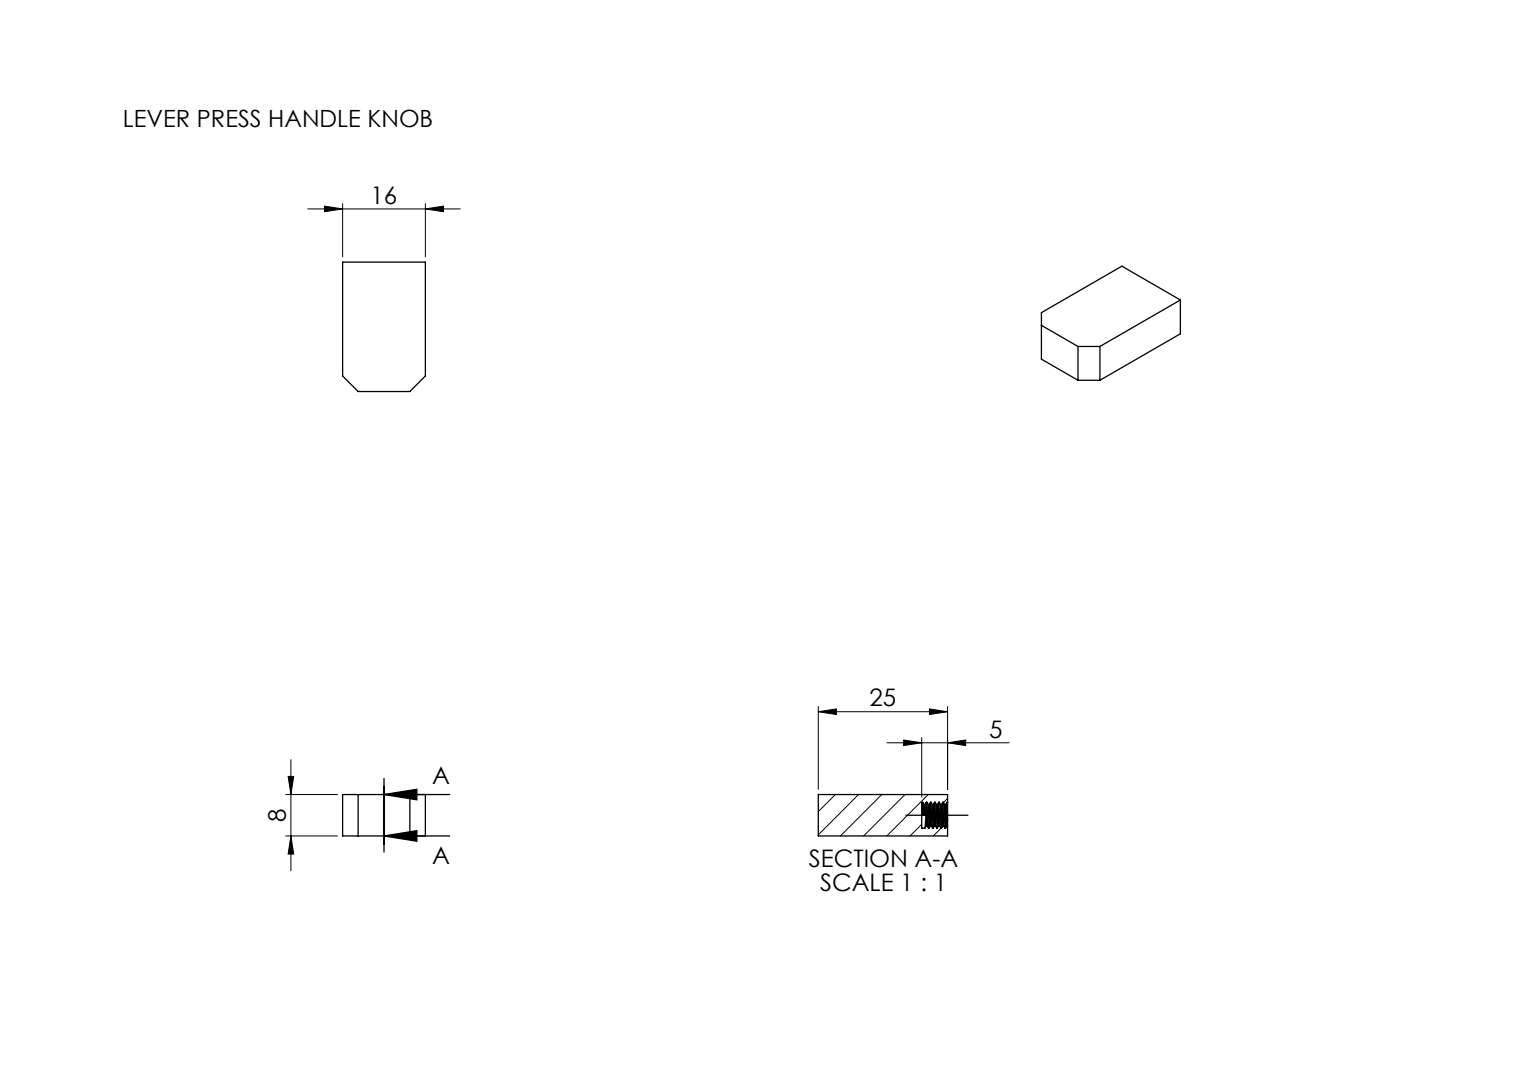
ISO-10303-21;
HEADER;
FILE_DESCRIPTION (('STEP AP214'),
    '1' );
FILE_NAME ('Lever Press Handle Knob.step',
    '2026-10-08T14:41:38',
    ( '' ),
    ( '' ),
    'SwSTEP 2.0',
    'SolidWorks 2026',
    '' );
FILE_SCHEMA (( 'AUTOMOTIVE_DESIGN' ));
ENDSEC;

DATA;
#12=LINE ( 'NONE', #3049, #2216 ) ;
#27=MECHANICAL_DESIGN_GEOMETRIC_PRESENTATION_REPRESENTATION('',(#18516),#10981);
#30=CARTESIAN_POINT ( 'NONE',  ( 2.500000000000001776, 64.00000000000000000, 49.99999999999999289 ) ) ;
#45=CARTESIAN_POINT ( 'NONE',  ( 4.592425496802577917E-16, 61.50000000000000000, 46.19999999999999574 ) ) ;
#69=CARTESIAN_POINT ( 'NONE',  ( 2.066987300000001859, 63.14382582708704916, 46.10000000109246798 ) ) ;
#77=ORIENTED_EDGE ( 'NONE', *, *, #16848, .F. ) ;
#82=CARTESIAN_POINT ( 'NONE',  ( 2.500000000000006661, 65.03553390593272354, 48.04999999999999716 ) ) ;
#83=CARTESIAN_POINT ( 'NONE',  ( 2.066987300000001859, 64.85617417291294373, 46.80000000109246372 ) ) ;
#85=EDGE_LOOP ( 'NONE', ( #12730, #3911, #462, #6972, #16450, #10959, #3705, #8319, #7529, #13845, #6781, #19380, #3029, #10375 ) ) ;
#92=CARTESIAN_POINT ( 'NONE',  ( -2.066987300000001415, 63.14382582708705627, 46.60000000109246088 ) ) ;
#105=CARTESIAN_POINT ( 'NONE',  ( 2.500000000000002220, 62.96446609406726225, 47.25000000218494023 ) ) ;
#113=DIRECTION ( 'NONE',  ( -0.000000000000000000, -0.000000000000000000, -1.000000000000000000 ) ) ;
#135=CARTESIAN_POINT ( 'NONE',  ( 0.000000000000000000, 64.00000000000000000, 49.99999999999999289 ) ) ;
#139=CARTESIAN_POINT ( 'NONE',  ( -2.500000000000001776, 64.00000000000000000, 46.79999999999999716 ) ) ;
#140=CARTESIAN_POINT ( 'NONE',  ( 4.592425496802577917E-16, 61.50000000000000000, 46.99999999999999289 ) ) ;
#161=CARTESIAN_POINT ( 'NONE',  ( 1.461580736456473906, 62.53841926354353120, 45.25000000109247367 ) ) ;
#162=CARTESIAN_POINT ( 'NONE',  ( -1.461580736456473906, 65.46158073645646880, 49.65000000109246514 ) ) ;
#179=DIRECTION ( 'NONE',  ( -0.000000000000000000, -0.000000000000000000, -1.000000000000000000 ) ) ;
#180=CARTESIAN_POINT ( 'NONE',  ( -2.066987300000001415, 64.00000000000000000, 46.35000000109246798 ) ) ;
#188=CARTESIAN_POINT ( 'NONE',  ( 2.066987300000001859, 64.85617417291294373, 46.20000000109247651 ) ) ;
#189=EDGE_CURVE ( 'NONE', #14847, #7431, #12616, .T. ) ;
#229=CARTESIAN_POINT ( 'NONE',  ( 1.767766952966369987, 65.76776695296638309, 45.69999999999999574 ) ) ;
#245=CARTESIAN_POINT ( 'NONE',  ( -0.8996865886453131456, 66.25031470727165583, 44.99999999999998579 ) ) ;
#257=CARTESIAN_POINT ( 'NONE',  ( -2.066987300000001415, 63.14382582708705627, 47.40000000109247225 ) ) ;
#270=CARTESIAN_POINT ( 'NONE',  ( 2.066987300000001415, 64.00000000000000000, 47.55000000109247082 ) ) ;
#271=ORIENTED_EDGE ( 'NONE', *, *, #18253, .T. ) ;
#278=CARTESIAN_POINT ( 'NONE',  ( -2.066987300000000971, 63.14382582708704916, 48.00000000109246656 ) ) ;
#296=CARTESIAN_POINT ( 'NONE',  ( 1.767766952966370653, 62.23223304703363112, 47.20000000218494307 ) ) ;
#316=CARTESIAN_POINT ( 'NONE',  ( 2.500000000000001776, 64.00000000000000000, 46.50000000218494733 ) ) ;
#331=AXIS2_PLACEMENT_3D ( 'NONE', #17063, #3625, #15585 ) ;
#334=LINE ( 'NONE', #13649, #1223 ) ;
#335=DIRECTION ( 'NONE',  ( -1.000000000000000000, 0.000000000000000000, 0.000000000000000000 ) ) ;
#345=AXIS2_PLACEMENT_3D ( 'NONE', #135, #15137, #1704 ) ;
#360=CARTESIAN_POINT ( 'NONE',  ( -1.265664690411616068E-16, 66.06698730000000808, 46.35000000109246798 ) ) ;
#373=CARTESIAN_POINT ( 'NONE',  ( -2.500000000000001776, 64.00000000000000000, 48.39999999999999858 ) ) ;
#374=CARTESIAN_POINT ( 'NONE',  ( 3.796994071234847710E-16, 61.93301269999999903, 47.35000000109246798 ) ) ;
#380=DIRECTION ( 'NONE',  ( -0.000000000000000000, -0.000000000000000000, -1.000000000000000000 ) ) ;
#382=CARTESIAN_POINT ( 'NONE',  ( -2.066987300000001415, 64.85617417291294373, 49.50000000109246656 ) ) ;
#385=CARTESIAN_POINT ( 'NONE',  ( 0.8561741729129460632, 66.06698729999999387, 45.50000000109247367 ) ) ;
#388=CARTESIAN_POINT ( 'NONE',  ( 2.500000000000001776, 64.00000000000000000, 47.30000000218494449 ) ) ;
#390=EDGE_LOOP ( 'NONE', ( #5193, #765, #2617, #19104 ) ) ;
#391=EDGE_LOOP ( 'NONE', ( #18321, #5980, #17279, #6106, #2334 ) ) ;
#405=CARTESIAN_POINT ( 'NONE',  ( 2.500000000000001776, 64.00000000000000000, 45.59999999999999432 ) ) ;
#410=CARTESIAN_POINT ( 'NONE',  ( 0.8561741729129472844, 61.93301270000000613, 48.20000000109248361 ) ) ;
#429=LINE ( 'NONE', #4946, #12185 ) ;
#438=CARTESIAN_POINT ( 'NONE',  ( -2.500000000000001776, 64.00000000000000000, 47.70000000218494307 ) ) ;
#455=CARTESIAN_POINT ( 'NONE',  ( -1.461580736456473906, 65.46158073645646880, 48.05000000109247082 ) ) ;
#462=ORIENTED_EDGE ( 'NONE', *, *, #8308, .F. ) ;
#467=CARTESIAN_POINT ( 'NONE',  ( -2.066987300000001859, 64.85617417291294373, 47.90000000109247225 ) ) ;
#470=CARTESIAN_POINT ( 'NONE',  ( -2.500000000000011546, 65.03553390593272354, 46.05000000218494449 ) ) ;
#473=CARTESIAN_POINT ( 'NONE',  ( 3.796994071234847710E-16, 61.93301269999999903, 48.95000000109246940 ) ) ;
#481=EDGE_LOOP ( 'NONE', ( #15484, #1248, #5355, #15133 ) ) ;
#491=DIRECTION ( 'NONE',  ( -1.000000000000000000, -0.000000000000000000, -0.000000000000000000 ) ) ;
#531=CARTESIAN_POINT ( 'NONE',  ( 1.767766952966369987, 65.76776695296638309, 46.49999999999999289 ) ) ;
#535=VERTEX_POINT ( 'NONE', #8772 ) ;
#548=DIRECTION ( 'NONE',  ( -1.000000000000000000, 0.000000000000000000, 0.000000000000000000 ) ) ;
#550=CARTESIAN_POINT ( 'NONE',  ( -1.265664690411616068E-16, 66.06698730000000808, 47.15000000109247225 ) ) ;
#566=CARTESIAN_POINT ( 'NONE',  ( -2.066987300000001415, 64.85617417291294373, 47.90000000109247225 ) ) ;
#568=LINE ( 'NONE', #6369, #960 ) ;
#574=VERTEX_POINT ( 'NONE', #10335 ) ;
#581=VECTOR ( 'NONE', #2799, 1000.000000000000000 ) ;
#595=CARTESIAN_POINT ( 'NONE',  ( 0.8561741729129460632, 66.06698729999999387, 47.70000000109248361 ) ) ;
#597=CARTESIAN_POINT ( 'NONE',  ( -2.066987300000000971, 63.14382582708704916, 48.20000000109247651 ) ) ;
#623=CARTESIAN_POINT ( 'NONE',  ( -1.767766952966370209, 65.76776695296638309, 45.09999999999999432 ) ) ;
#637=FACE_OUTER_BOUND ( 'NONE', #1554, .T. ) ;
#647=CARTESIAN_POINT ( 'NONE',  ( -0.8561741729129465073, 61.93301270000000613, 48.30000000109247082 ) ) ;
#663=VERTEX_POINT ( 'NONE', #14958 ) ;
#669=CARTESIAN_POINT ( 'NONE',  ( 2.066987300000001859, 63.14382582708704916, 49.10000000109246088 ) ) ;
#677=VERTEX_POINT ( 'NONE', #10628 ) ;
#680=( NAMED_UNIT ( * ) PLANE_ANGLE_UNIT ( ) SI_UNIT ( $, .RADIAN. ) );
#682=ORIENTED_EDGE ( 'NONE', *, *, #6769, .F. ) ;
#683=EDGE_LOOP ( 'NONE', ( #8801, #8791, #6089, #8526 ) ) ;
#687=CARTESIAN_POINT ( 'NONE',  ( 2.500000000000001776, 64.00000000000000000, 47.30000000218494449 ) ) ;
#699=LINE ( 'NONE', #15785, #15320 ) ;
#700=CARTESIAN_POINT ( 'NONE',  ( -1.265664690411616068E-16, 66.06698730000000808, 48.55000000109247082 ) ) ;
#701=CARTESIAN_POINT ( 'NONE',  ( -2.066987300000001415, 64.85617417291294373, 49.70000000109247651 ) ) ;
#740=CARTESIAN_POINT ( 'NONE',  ( -2.500000000000001776, 64.00000000000000000, 48.50000000218494023 ) ) ;
#741=CARTESIAN_POINT ( 'NONE',  ( 2.066987300000001859, 64.85617417291294373, 46.20000000109247651 ) ) ;
#753=CARTESIAN_POINT ( 'NONE',  ( -0.8561741729129466183, 61.93301270000000613, 45.70000000109248361 ) ) ;
#761=CARTESIAN_POINT ( 'NONE',  ( -2.499999999999998668, 62.96446609406726225, 47.64999999999999858 ) ) ;
#765=ORIENTED_EDGE ( 'NONE', *, *, #8549, .F. ) ;
#772=CARTESIAN_POINT ( 'NONE',  ( -2.500000000000001776, 64.00000000000000000, 48.50000000218494023 ) ) ;
#784=CARTESIAN_POINT ( 'NONE',  ( 2.066987300000002303, 63.14382582708705627, 45.10000000109246798 ) ) ;
#786=CARTESIAN_POINT ( 'NONE',  ( 1.461580736456473906, 62.53841926354353120, 48.45000000109246940 ) ) ;
#812=DIRECTION ( 'NONE',  ( 0.7071067811865463515, 0.000000000000000000, -0.7071067811865487940 ) ) ;
#832=CARTESIAN_POINT ( 'NONE',  ( -2.500000000000000888, 62.96446609406726935, 48.44999999999999574 ) ) ;
#839=CARTESIAN_POINT ( 'NONE',  ( 2.500000000000001776, 64.00000000000000000, 48.79999999999999716 ) ) ;
#845=CARTESIAN_POINT ( 'NONE',  ( -1.265664690411616068E-16, 66.06698730000000808, 46.95000000109246940 ) ) ;
#847=EDGE_CURVE ( 'NONE', #14186, #5501, #5607, .T. ) ;
#863=CARTESIAN_POINT ( 'NONE',  ( -1.530808498934192803E-16, 66.50000000000000000, 49.10000000218494165 ) ) ;
#875=CARTESIAN_POINT ( 'NONE',  ( -1.461580736456473906, 65.46158073645646880, 47.05000000109247082 ) ) ;
#879=LINE ( 'NONE', #8340, #1099 ) ;
#907=ADVANCED_FACE ( 'NONE', ( #15824 ), #16023, .F. ) ;
#926=CARTESIAN_POINT ( 'NONE',  ( 2.500000000000002220, 62.96446609406726935, 49.54999999999999716 ) ) ;
#942=CARTESIAN_POINT ( 'NONE',  ( 2.066987300000001415, 64.00000000000000000, 47.55000000109247082 ) ) ;
#957=EDGE_CURVE ( 'NONE', #15953, #1682, #18392, .T. ) ;
#960=VECTOR ( 'NONE', #4995, 1000.000000000000000 ) ;
#962=CARTESIAN_POINT ( 'NONE',  ( -1.767766952966369765, 62.23223304703363112, 47.00000000218494733 ) ) ;
#976=CARTESIAN_POINT ( 'NONE',  ( 2.066987300000001415, 64.00000000000000000, 45.95000000109246940 ) ) ;
#980=CARTESIAN_POINT ( 'NONE',  ( 1.145374997815830520, 62.22070308213160672, 44.99999999999998579 ) ) ;
#986=ORIENTED_EDGE ( 'NONE', *, *, #5520, .T. ) ;
#994=CIRCLE ( 'NONE', #16652, 2.500000000000001776 ) ;
#1004=CARTESIAN_POINT ( 'NONE',  ( -2.066987300000001415, 64.00000000000000000, 49.55000000109247082 ) ) ;
#1028=CARTESIAN_POINT ( 'NONE',  ( 1.035533905932738197, 66.50000000000000000, 48.94999999999999574 ) ) ;
#1040=CARTESIAN_POINT ( 'NONE',  ( 2.066987300000001859, 63.14382582708704916, 45.90000000109247225 ) ) ;
#1055=CARTESIAN_POINT ( 'NONE',  ( 1.035533905932738197, 66.50000000000000000, 46.65000000218494591 ) ) ;
#1067=CARTESIAN_POINT ( 'NONE',  ( 3.796994071234847710E-16, 61.93301269999999903, 46.55000000109247082 ) ) ;
#1099=VECTOR ( 'NONE', #2541, 1000.000000000000000 ) ;
#1104=CARTESIAN_POINT ( 'NONE',  ( -1.265664690411616068E-16, 66.06698730000000808, 44.55000000109247082 ) ) ;
#1120=CARTESIAN_POINT ( 'NONE',  ( 2.066987300000001859, 64.85617417291294373, 45.40000000109246514 ) ) ;
#1136=CARTESIAN_POINT ( 'NONE',  ( -2.066987300000001415, 64.00000000000000000, 46.35000000109246798 ) ) ;
#1139=CARTESIAN_POINT ( 'NONE',  ( 2.066987300000001859, 63.14382582708704916, 47.70000000109246940 ) ) ;
#1154=CARTESIAN_POINT ( 'NONE',  ( 0.8561741729129472844, 61.93301270000000613, 49.00000000109246656 ) ) ;
#1164=CARTESIAN_POINT ( 'NONE',  ( 0.8561741729129460632, 66.06698729999999387, 46.90000000109247225 ) ) ;
#1194=DIRECTION ( 'NONE',  ( -1.000000000000000000, 0.000000000000000000, 0.000000000000000000 ) ) ;
#1210=EDGE_CURVE ( 'NONE', #9690, #15813, #699, .T. ) ;
#1213=CARTESIAN_POINT ( 'NONE',  ( 2.500000000000002220, 62.96446609406726935, 45.54999999999999716 ) ) ;
#1223=VECTOR ( 'NONE', #16705, 1000.000000000000000 ) ;
#1234=CARTESIAN_POINT ( 'NONE',  ( -2.066987300000001415, 64.00000000000000000, 48.95000000109246940 ) ) ;
#1248=ORIENTED_EDGE ( 'NONE', *, *, #14177, .T. ) ;
#1255=CARTESIAN_POINT ( 'NONE',  ( -1.035533905932738863, 61.50000000000000000, 45.45000000218495018 ) ) ;
#1259=VERTEX_POINT ( 'NONE', #9699 ) ;
#1266=CARTESIAN_POINT ( 'NONE',  ( 2.066987300000002303, 63.14382582708705627, 48.50000000109246656 ) ) ;
#1323=CARTESIAN_POINT ( 'NONE',  ( -2.500000000000001776, 65.03553390593273775, 45.14999999999999858 ) ) ;
#1330=CARTESIAN_POINT ( 'NONE',  ( -2.169199425089220146, 64.10592246629431656, 45.00000000000000000 ) ) ;
#1347=SHAPE_REPRESENTATION_RELATIONSHIP ( 'NONE' , 'NONE' ,  #15288, #12018 ) ;
#1355=CARTESIAN_POINT ( 'NONE',  ( 1.767766952966369987, 65.76776695296638309, 45.80000000218493739 ) ) ;
#1367=CARTESIAN_POINT ( 'NONE',  ( 3.796994071234847710E-16, 61.93301269999999903, 47.55000000109247082 ) ) ;
#1387=CARTESIAN_POINT ( 'NONE',  ( 8.000000000000014211, 60.00000000000000711, 45.00000000000000000 ) ) ;
#1396=ORIENTED_EDGE ( 'NONE', *, *, #6504, .F. ) ;
#1417=CARTESIAN_POINT ( 'NONE',  ( 4.592425496802577917E-16, 61.50000000000000000, 47.79999999999999716 ) ) ;
#1437=CARTESIAN_POINT ( 'NONE',  ( -2.066987300000001415, 64.85617417291294373, 45.70000000109248361 ) ) ;
#1454=CARTESIAN_POINT ( 'NONE',  ( 4.592425496802577917E-16, 61.50000000000000000, 44.70000000218494307 ) ) ;
#1466=CARTESIAN_POINT ( 'NONE',  ( -2.066987300000001415, 63.14382582708705627, 47.40000000109247225 ) ) ;
#1470=CARTESIAN_POINT ( 'NONE',  ( -7.999999999999986677, 68.00000000000000000, 66.99999999999997158 ) ) ;
#1477=ORIENTED_EDGE ( 'NONE', *, *, #18253, .F. ) ;
#1494=CARTESIAN_POINT ( 'NONE',  ( -2.499999999999992006, 62.96446609406726225, 46.15000000218496012 ) ) ;
#1508=ORIENTED_EDGE ( 'NONE', *, *, #15852, .T. ) ;
#1519=CARTESIAN_POINT ( 'NONE',  ( 1.035533905932738197, 66.50000000000000000, 47.34999999999999432 ) ) ;
#1521=ORIENTED_EDGE ( 'NONE', *, *, #17939, .T. ) ;
#1526=CARTESIAN_POINT ( 'NONE',  ( -1.909647267044692676, 63.20899822134837365, 45.00000000000000000 ) ) ;
#1540=ORIENTED_EDGE ( 'NONE', *, *, #6380, .F. ) ;
#1552=CARTESIAN_POINT ( 'NONE',  ( 0.8561741729129460632, 66.06698729999999387, 49.30000000109246372 ) ) ;
#1554=EDGE_LOOP ( 'NONE', ( #9866, #4096, #2330, #1508, #682, #6069 ) ) ;
#1561=CARTESIAN_POINT ( 'NONE',  ( -0.8561741729129465073, 61.93301270000000613, 46.70000000109248361 ) ) ;
#1588=FACE_OUTER_BOUND ( 'NONE', #481, .T. ) ;
#1604=CARTESIAN_POINT ( 'NONE',  ( -2.500000000000001776, 64.00000000000000000, 47.70000000218494307 ) ) ;
#1621=CARTESIAN_POINT ( 'NONE',  ( -1.530808498934192803E-16, 66.50000000000000000, 48.19999999999999574 ) ) ;
#1642=CARTESIAN_POINT ( 'NONE',  ( -2.066987300000001415, 64.00000000000000000, 46.55000000109247082 ) ) ;
#1645=FACE_OUTER_BOUND ( 'NONE', #683, .T. ) ;
#1656=CARTESIAN_POINT ( 'NONE',  ( 3.796994071234847710E-16, 61.93301269999999903, 48.15000000109247225 ) ) ;
#1660=CARTESIAN_POINT ( 'NONE',  ( 1.767766952966369987, 65.76776695296638309, 45.80000000218493739 ) ) ;
#1665=CARTESIAN_POINT ( 'NONE',  ( 2.066987300000002303, 63.14382582708705627, 46.90000000109247225 ) ) ;
#1667=CARTESIAN_POINT ( 'NONE',  ( -1.767766952966370209, 65.76776695296638309, 47.60000000218494165 ) ) ;
#1682=VERTEX_POINT ( 'NONE', #9102 ) ;
#1687=CARTESIAN_POINT ( 'NONE',  ( -2.500000000000001776, 64.00000000000000000, 46.10000000218494165 ) ) ;
#1704=DIRECTION ( 'NONE',  ( -1.000000000000000000, 0.000000000000000000, 0.000000000000000000 ) ) ;
#1731=CARTESIAN_POINT ( 'NONE',  ( 0.8561741729129471734, 61.93301270000000613, 46.00000000109246656 ) ) ;
#1732=CARTESIAN_POINT ( 'NONE',  ( -0.8561741729129465073, 61.93301270000000613, 46.70000000109248361 ) ) ;
#1733=DIRECTION ( 'NONE',  ( -0.7071067811865463515, 0.000000000000000000, -0.7071067811865487940 ) ) ;
#1747=CARTESIAN_POINT ( 'NONE',  ( 1.461580736456473684, 65.46158073645646880, 46.85000000109246798 ) ) ;
#1754=FACE_OUTER_BOUND ( 'NONE', #4883, .T. ) ;
#1791=AXIS2_PLACEMENT_3D ( 'NONE', #13713, #4815, #7646 ) ;
#1816=EDGE_CURVE ( 'NONE', #6405, #8644, #12331, .T. ) ;
#1827=DIRECTION ( 'NONE',  ( -0.000000000000000000, -0.000000000000000000, -1.000000000000000000 ) ) ;
#1828=CARTESIAN_POINT ( 'NONE',  ( -1.530808498934192803E-16, 66.50000000000000000, 48.30000000218494449 ) ) ;
#1829=CARTESIAN_POINT ( 'NONE',  ( 3.796994071234847710E-16, 61.93301269999999903, 49.15000000109246514 ) ) ;
#1841=CARTESIAN_POINT ( 'NONE',  ( -2.066987300000001859, 64.85617417291294373, 46.30000000109247082 ) ) ;
#1855=CARTESIAN_POINT ( 'NONE',  ( -1.035533905932738863, 61.50000000000000000, 45.45000000218494307 ) ) ;
#1886=CARTESIAN_POINT ( 'NONE',  ( 0.000000000000000000, 64.00000000000000000, 49.99999999999999289 ) ) ;
#1897=( BOUNDED_CURVE ( )  B_SPLINE_CURVE ( 2, ( #3126, #18429, #1667, #13901, #3522, #10664, #16664, #3229, #388 ),
 .UNSPECIFIED., .F., .F. ) 
 B_SPLINE_CURVE_WITH_KNOTS ( ( 3, 2, 2, 2, 3 ),
 ( 0.2857142857142859205, 0.3035714285714287142, 0.3214285714285715634, 0.3392857142857143571, 0.3571428571428571508 ),
 .UNSPECIFIED. ) 
 CURVE ( )  GEOMETRIC_REPRESENTATION_ITEM ( )  RATIONAL_B_SPLINE_CURVE ( ( 0.9999999999999990008, 0.9238795325112877377, 1.000000000000000000, 0.9238795325112867385, 1.000000000000000000, 0.9238795325112867385, 1.000000000000000000, 0.9238795325112867385, 1.000000000000000000 ) ) 
 REPRESENTATION_ITEM ( '' )  );
#1933=CARTESIAN_POINT ( 'NONE',  ( -1.461580736456473906, 65.46158073645646880, 48.85000000109246798 ) ) ;
#1935=ORIENTED_EDGE ( 'NONE', *, *, #14860, .F. ) ;
#1946=CARTESIAN_POINT ( 'NONE',  ( 2.066987300000001415, 64.00000000000000000, 45.95000000109246940 ) ) ;
#1953=CARTESIAN_POINT ( 'NONE',  ( 1.461580736456473906, 62.53841926354353120, 45.25000000109247367 ) ) ;
#1961=ORIENTED_EDGE ( 'NONE', *, *, #10797, .F. ) ;
#1980=CARTESIAN_POINT ( 'NONE',  ( -1.461580736456473906, 65.46158073645646880, 48.65000000109247225 ) ) ;
#2014=CARTESIAN_POINT ( 'NONE',  ( 2.499999999999996891, 62.96446609406726225, 47.14999999999999147 ) ) ;
#2020=CARTESIAN_POINT ( 'NONE',  ( -2.066987300000001415, 64.00000000000000000, 47.35000000109246798 ) ) ;
#2030=CARTESIAN_POINT ( 'NONE',  ( 0.7910017786515960436, 62.09035273295529578, 44.99999999999998579 ) ) ;
#2033=CARTESIAN_POINT ( 'NONE',  ( -0.8561741729129461742, 66.06698729999999387, 47.00000000109247367 ) ) ;
#2037=CARTESIAN_POINT ( 'NONE',  ( 2.500000000000001776, 65.03553390593273775, 45.75000000218494733 ) ) ;
#2063=( NAMED_UNIT ( * ) SI_UNIT ( $, .STERADIAN. ) SOLID_ANGLE_UNIT ( ) );
#2066=ORIENTED_EDGE ( 'NONE', *, *, #14389, .F. ) ;
#2114=CARTESIAN_POINT ( 'NONE',  ( -1.767766952966369765, 62.23223304703363112, 46.89999999999999858 ) ) ;
#2121=CARTESIAN_POINT ( 'NONE',  ( 1.461580736456473906, 62.53841926354353120, 46.85000000109246798 ) ) ;
#2138=CARTESIAN_POINT ( 'NONE',  ( -2.500000000000001776, 64.00000000000000000, 49.99999999999999289 ) ) ;
#2139=CARTESIAN_POINT ( 'NONE',  ( -1.461580736456473906, 65.46158073645646880, 44.85000000109246798 ) ) ;
#2140=FACE_OUTER_BOUND ( 'NONE', #5028, .T. ) ;
#2152=CARTESIAN_POINT ( 'NONE',  ( -2.500000000000000888, 62.96446609406726935, 47.75000000218494023 ) ) ;
#2156=PRESENTATION_STYLE_ASSIGNMENT (( #12547 ) ) ;
#2165=CARTESIAN_POINT ( 'NONE',  ( 1.461580736456473684, 65.46158073645646880, 47.05000000109247082 ) ) ;
#2183=CARTESIAN_POINT ( 'NONE',  ( -2.500000000000001776, 64.00000000000000000, 45.30000000218493739 ) ) ;
#2200=VECTOR ( 'NONE', #3797, 1000.000000000000000 ) ;
#2211=CARTESIAN_POINT ( 'NONE',  ( -7.999999999999986677, 60.00000000000000711, 45.00000000000000000 ) ) ;
#2214=CARTESIAN_POINT ( 'NONE',  ( 1.767766952966370653, 62.23223304703363112, 48.69999999999999574 ) ) ;
#2216=VECTOR ( 'NONE', #9024, 1000.000000000000000 ) ;
#2232=CARTESIAN_POINT ( 'NONE',  ( -1.265664690411616068E-16, 66.06698730000000808, 45.35000000109246798 ) ) ;
#2240=ORIENTED_EDGE ( 'NONE', *, *, #2551, .T. ) ;
#2251=CARTESIAN_POINT ( 'NONE',  ( -2.500000000000001776, 65.03553390593273775, 49.25000000218494023 ) ) ;
#2263=CARTESIAN_POINT ( 'NONE',  ( 2.066987300000001415, 64.00000000000000000, 49.15000000109247225 ) ) ;
#2264=CARTESIAN_POINT ( 'NONE',  ( 0.8561741729129471734, 61.93301270000000613, 46.80000000109247082 ) ) ;
#2287=CARTESIAN_POINT ( 'NONE',  ( 11.00000000000002309, 68.00000000000000000, 63.99999999999994316 ) ) ;
#2293=EDGE_CURVE ( 'NONE', #6744, #15813, #4783, .T. ) ;
#2300=CARTESIAN_POINT ( 'NONE',  ( 2.500000000000001776, 64.00000000000000000, 46.50000000218494733 ) ) ;
#2305=CARTESIAN_POINT ( 'NONE',  ( 1.035533905932739751, 61.50000000000000000, 49.44999999999999574 ) ) ;
#2328=CARTESIAN_POINT ( 'NONE',  ( -1.035533905932738863, 61.50000000000000000, 47.74999999999999289 ) ) ;
#2330=ORIENTED_EDGE ( 'NONE', *, *, #15528, .F. ) ;
#2334=ORIENTED_EDGE ( 'NONE', *, *, #9822, .F. ) ;
#2341=CARTESIAN_POINT ( 'NONE',  ( -2.500000000000001776, 64.00000000000000000, 46.10000000218494165 ) ) ;
#2348=CARTESIAN_POINT ( 'NONE',  ( -1.909647267044692676, 63.20899822134837365, 45.00000000000000000 ) ) ;
#2351=CARTESIAN_POINT ( 'NONE',  ( -1.265664690411616068E-16, 66.06698730000000808, 49.55000000109247082 ) ) ;
#2353=CARTESIAN_POINT ( 'NONE',  ( -2.066987300000001415, 64.00000000000000000, 47.35000000109246798 ) ) ;
#2362=VERTEX_POINT ( 'NONE', #14169 ) ;
#2396=CARTESIAN_POINT ( 'NONE',  ( 1.035533905932738197, 66.50000000000000000, 49.75000000000000000 ) ) ;
#2410=CARTESIAN_POINT ( 'NONE',  ( -2.066987300000001415, 64.85617417291294373, 47.10000000109246798 ) ) ;
#2427=CARTESIAN_POINT ( 'NONE',  ( 2.500000000000002220, 62.96446609406726935, 48.05000000218494449 ) ) ;
#2440=CARTESIAN_POINT ( 'NONE',  ( 0.8561741729129472844, 61.93301270000000613, 46.60000000109246088 ) ) ;
#2443=CARTESIAN_POINT ( 'NONE',  ( 1.976658868803501834, 62.97126298013989754, 45.00000000000001421 ) ) ;
#2476=CARTESIAN_POINT ( 'NONE',  ( -2.066987300000001859, 64.85617417291294373, 44.70000000109248361 ) ) ;
#2482=CARTESIAN_POINT ( 'NONE',  ( 2.499999999999999112, 65.03553390593273775, 46.55000000218494449 ) ) ;
#2489=CARTESIAN_POINT ( 'NONE',  ( -2.066987300000001415, 63.14382582708705627, 45.80000000109246372 ) ) ;
#2506=CARTESIAN_POINT ( 'NONE',  ( 2.066987300000001415, 64.85617417291294373, 46.00000000109247367 ) ) ;
#2525=CARTESIAN_POINT ( 'NONE',  ( -2.500000000000000888, 62.96446609406726935, 46.95000000218495018 ) ) ;
#2537=CARTESIAN_POINT ( 'NONE',  ( 0.8561741729129460632, 66.06698729999999387, 46.10000000109246798 ) ) ;
#2541=DIRECTION ( 'NONE',  ( -0.7071067811865463515, 0.000000000000000000, 0.7071067811865487940 ) ) ;
#2551=EDGE_CURVE ( 'NONE', #10838, #14706, #8107, .T. ) ;
#2564=CARTESIAN_POINT ( 'NONE',  ( -2.283493650000001818, 64.00000000000000000, 49.87500000054622973 ) ) ;
#2568=DIRECTION ( 'NONE',  ( -0.8660254037844385966, 0.000000000000000000, 0.5000000000000001110 ) ) ;
#2576=CARTESIAN_POINT ( 'NONE',  ( -0.8561741729129465073, 61.93301270000000613, 44.90000000109247225 ) ) ;
#2588=CARTESIAN_POINT ( 'NONE',  ( 0.8561741729129472844, 61.93301270000000613, 46.00000000109245946 ) ) ;
#2601=CARTESIAN_POINT ( 'NONE',  ( -2.066987300000000971, 63.14382582708704916, 45.60000000109246798 ) ) ;
#2610=ORIENTED_EDGE ( 'NONE', *, *, #17643, .F. ) ;
#2615=CARTESIAN_POINT ( 'NONE',  ( 0.8561741729129472844, 61.93301270000000613, 48.20000000109248361 ) ) ;
#2617=ORIENTED_EDGE ( 'NONE', *, *, #13137, .F. ) ;
#2626=CARTESIAN_POINT ( 'NONE',  ( 2.066987300000001859, 64.85617417291294373, 45.20000000109248361 ) ) ;
#2645=EDGE_CURVE ( 'NONE', #677, #16168, #16710, .T. ) ;
#2688=CARTESIAN_POINT ( 'NONE',  ( -1.767766952966369765, 62.23223304703363112, 45.29999999999999005 ) ) ;
#2705=CARTESIAN_POINT ( 'NONE',  ( 2.066987300000001415, 64.00000000000000000, 46.95000000109246940 ) ) ;
#2706=DIRECTION ( 'NONE',  ( 0.7071067811865487940, 1.226634733346701480E-15, 0.7071067811865462405 ) ) ;
#2721=CARTESIAN_POINT ( 'NONE',  ( -1.767766952966369765, 62.23223304703363112, 45.40000000218494591 ) ) ;
#2732=CARTESIAN_POINT ( 'NONE',  ( -2.066987300000001415, 64.00000000000000000, 49.75000000109246656 ) ) ;
#2779=CARTESIAN_POINT ( 'NONE',  ( -2.500000000000001776, 65.03553390593273775, 46.74999999999999289 ) ) ;
#2780=CARTESIAN_POINT ( 'NONE',  ( 1.035533905932739751, 61.50000000000000000, 46.24999999999998579 ) ) ;
#2786=EDGE_CURVE ( 'NONE', #18046, #15953, #15628, .T. ) ;
#2799=DIRECTION ( 'NONE',  ( 0.000000000000000000, 0.000000000000000000, 1.000000000000000000 ) ) ;
#2800=DIRECTION ( 'NONE',  ( -1.000000000000000000, 0.000000000000000000, 0.000000000000000000 ) ) ;
#2802=CARTESIAN_POINT ( 'NONE',  ( -1.461580736456473906, 65.46158073645646880, 48.85000000109246798 ) ) ;
#2806=ORIENTED_EDGE ( 'NONE', *, *, #19318, .F. ) ;
#2818=CARTESIAN_POINT ( 'NONE',  ( -2.500000000000001776, 65.03553390593273775, 46.05000000218494449 ) ) ;
#2828=CARTESIAN_POINT ( 'NONE',  ( 0.8561741729129472844, 61.93301270000000613, 47.60000000109246798 ) ) ;
#2847=DIRECTION ( 'NONE',  ( -1.000000000000000000, 0.000000000000000000, 0.000000000000000000 ) ) ;
#2848=ORIENTED_EDGE ( 'NONE', *, *, #957, .F. ) ;
#2882=CARTESIAN_POINT ( 'NONE',  ( -1.767766952966370209, 65.76776695296638309, 47.49999999999999289 ) ) ;
#2904=CARTESIAN_POINT ( 'NONE',  ( -0.8561741729129461742, 66.06698729999999387, 49.60000000109246798 ) ) ;
#2918=CARTESIAN_POINT ( 'NONE',  ( -1.265664690411616068E-16, 66.06698730000000808, 48.55000000109247082 ) ) ;
#2926=CARTESIAN_POINT ( 'NONE',  ( -0.8561741729129461742, 66.06698729999999387, 48.80000000109247082 ) ) ;
#2927=EDGE_CURVE ( 'NONE', #3230, #15072, #9595, .T. ) ;
#2951=DIRECTION ( 'NONE',  ( -0.000000000000000000, -0.000000000000000000, -1.000000000000000000 ) ) ;
#2953=CARTESIAN_POINT ( 'NONE',  ( -1.035533905932738863, 61.50000000000000000, 46.25000000218494733 ) ) ;
#2963=CARTESIAN_POINT ( 'NONE',  ( -1.530808498934192803E-16, 66.50000000000000000, 45.79999999999999005 ) ) ;
#2973=FACE_OUTER_BOUND ( 'NONE', #9281, .T. ) ;
#2976=CARTESIAN_POINT ( 'NONE',  ( 1.767766952966370653, 62.23223304703363112, 47.89999999999999858 ) ) ;
#2983=CARTESIAN_POINT ( 'NONE',  ( -0.1886580908559672143, 66.48422237085870279, 45.00000000000000711 ) ) ;
#2995=DIRECTION ( 'NONE',  ( 0.8660254037844385966, 0.000000000000000000, 0.5000000000000001110 ) ) ;
#2996=CARTESIAN_POINT ( 'NONE',  ( 2.066987300000001415, 64.00000000000000000, 45.35000000109246798 ) ) ;
#3011=CARTESIAN_POINT ( 'NONE',  ( -1.767766952966369765, 62.23223304703363112, 48.60000000218494165 ) ) ;
#3015=CARTESIAN_POINT ( 'NONE',  ( -1.767766952966370209, 65.76776695296638309, 44.40000000218493881 ) ) ;
#3020=ORIENTED_EDGE ( 'NONE', *, *, #8179, .F. ) ;
#3025=CARTESIAN_POINT ( 'NONE',  ( 2.066987300000001415, 64.00000000000000000, 47.75000000109246656 ) ) ;
#3029=ORIENTED_EDGE ( 'NONE', *, *, #17851, .T. ) ;
#3030=ORIENTED_EDGE ( 'NONE', *, *, #15550, .T. ) ;
#3043=ADVANCED_FACE ( 'NONE', ( #14207 ), #10769, .T. ) ;
#3046=ORIENTED_EDGE ( 'NONE', *, *, #10797, .T. ) ;
#3049=CARTESIAN_POINT ( 'NONE',  ( 8.000000000000000000, 68.00000000000000000, 45.00000000000000000 ) ) ;
#3075=CARTESIAN_POINT ( 'NONE',  ( 2.500000000000001776, 64.00000000000000000, 47.99999999999999289 ) ) ;
#3076=CARTESIAN_POINT ( 'NONE',  ( -2.500000000000001776, 64.00000000000000000, 49.99999999999999289 ) ) ;
#3094=CARTESIAN_POINT ( 'NONE',  ( -1.461580736456473462, 62.53841926354353120, 46.65000000109247225 ) ) ;
#3109=CARTESIAN_POINT ( 'NONE',  ( 2.500000000000001776, 64.00000000000000000, 48.90000000218494591 ) ) ;
#3114=CARTESIAN_POINT ( 'NONE',  ( 2.066987300000001415, 64.00000000000000000, 46.75000000109247367 ) ) ;
#3123=CARTESIAN_POINT ( 'NONE',  ( 0.8561741729129460632, 66.06698729999999387, 46.30000000109247082 ) ) ;
#3126=CARTESIAN_POINT ( 'NONE',  ( -2.500000000000001776, 64.00000000000000000, 47.70000000218494307 ) ) ;
#3149=CARTESIAN_POINT ( 'NONE',  ( -2.500000000000001776, 64.00000000000000000, 49.99999999999999289 ) ) ;
#3162=ORIENTED_EDGE ( 'NONE', *, *, #13703, .F. ) ;
#3180=DIRECTION ( 'NONE',  ( 1.000000000000000000, 0.000000000000000000, -0.000000000000000000 ) ) ;
#3184=EDGE_CURVE ( 'NONE', #10801, #17922, #3906, .T. ) ;
#3196=CARTESIAN_POINT ( 'NONE',  ( -7.999999999999986677, 60.00000000000000711, 45.00000000000000000 ) ) ;
#3203=CARTESIAN_POINT ( 'NONE',  ( 2.066987300000001415, 64.00000000000000000, 46.15000000109247225 ) ) ;
#3208=ORIENTED_EDGE ( 'NONE', *, *, #12727, .T. ) ;
#3219=CARTESIAN_POINT ( 'NONE',  ( -2.066987300000001415, 63.14382582708705627, 45.60000000109246088 ) ) ;
#3225=CARTESIAN_POINT ( 'NONE',  ( 2.066987300000001415, 64.85617417291294373, 48.40000000109247225 ) ) ;
#3227=CARTESIAN_POINT ( 'NONE',  ( 1.461580736456473906, 62.53841926354353120, 46.05000000109246372 ) ) ;
#3229=CARTESIAN_POINT ( 'NONE',  ( 2.500000000000001776, 65.03553390593273775, 47.35000000218494165 ) ) ;
#3230=VERTEX_POINT ( 'NONE', #17522 ) ;
#3245=CARTESIAN_POINT ( 'NONE',  ( -2.499999999999996003, 62.96446609406726225, 45.25000000000000000 ) ) ;
#3250=DIRECTION ( 'NONE',  ( -0.000000000000000000, -0.000000000000000000, -1.000000000000000000 ) ) ;
#3255=ADVANCED_FACE ( 'NONE', ( #11528 ), #8258, .F. ) ;
#3297=EDGE_CURVE ( 'NONE', #574, #8644, #10230, .T. ) ;
#3302=CARTESIAN_POINT ( 'NONE',  ( 1.767766952966369987, 65.76776695296638309, 48.20000000218494307 ) ) ;
#3303=CARTESIAN_POINT ( 'NONE',  ( -1.265664690411616068E-16, 66.06698730000000808, 47.95000000109246940 ) ) ;
#3317=CARTESIAN_POINT ( 'NONE',  ( -2.500000000000001776, 64.00000000000000000, 49.99999999999999289 ) ) ;
#3318=CARTESIAN_POINT ( 'NONE',  ( 1.461580736456473684, 65.46158073645646880, 45.25000000109247367 ) ) ;
#3323=ORIENTED_EDGE ( 'NONE', *, *, #13137, .T. ) ;
#3337=ORIENTED_EDGE ( 'NONE', *, *, #1816, .F. ) ;
#3355=CARTESIAN_POINT ( 'NONE',  ( 1.461580736456473906, 62.53841926354353120, 49.05000000109247082 ) ) ;
#3376=LINE ( 'NONE', #3076, #14576 ) ;
#3392=CARTESIAN_POINT ( 'NONE',  ( -2.066987300000001859, 64.85617417291294373, 48.10000000109246798 ) ) ;
#3407=CARTESIAN_POINT ( 'NONE',  ( -2.066987300000001415, 64.00000000000000000, 47.15000000109247225 ) ) ;
#3408=ORIENTED_EDGE ( 'NONE', *, *, #1816, .T. ) ;
#3413=CARTESIAN_POINT ( 'NONE',  ( -1.265664690411616068E-16, 66.06698730000000808, 48.55000000109247082 ) ) ;
#3415=CARTESIAN_POINT ( 'NONE',  ( -0.8561741729129465073, 61.93301270000000613, 45.10000000109246798 ) ) ;
#3452=ORIENTED_EDGE ( 'NONE', *, *, #14948, .F. ) ;
#3473=CARTESIAN_POINT ( 'NONE',  ( -1.530808498934192803E-16, 66.50000000000000000, 45.00000000000000000 ) ) ;
#3476=ORIENTED_EDGE ( 'NONE', *, *, #6386, .F. ) ;
#3490=DIRECTION ( 'NONE',  ( 0.000000000000000000, 0.000000000000000000, 1.000000000000000000 ) ) ;
#3493=CARTESIAN_POINT ( 'NONE',  ( -1.461580736456473462, 62.53841926354353120, 47.45000000109246230 ) ) ;
#3511=CARTESIAN_POINT ( 'NONE',  ( -1.461580736456473906, 65.46158073645646880, 46.25000000109247367 ) ) ;
#3515=CARTESIAN_POINT ( 'NONE',  ( 1.035533905932738197, 66.50000000000000000, 45.85000000218494165 ) ) ;
#3519=EDGE_CURVE ( 'NONE', #7431, #4122, #10990, .T. ) ;
#3520=CARTESIAN_POINT ( 'NONE',  ( -1.461580736456473906, 65.46158073645646880, 45.65000000109247225 ) ) ;
#3522=CARTESIAN_POINT ( 'NONE',  ( -1.530808498934192803E-16, 66.50000000000000000, 47.50000000218494023 ) ) ;
#3536=EDGE_CURVE ( 'NONE', #5700, #574, #13446, .T. ) ;
#3544=CARTESIAN_POINT ( 'NONE',  ( -1.461580736456473906, 65.46158073645646880, 47.85000000109246798 ) ) ;
#3586=CARTESIAN_POINT ( 'NONE',  ( 1.461580736456473906, 62.53841926354353120, 49.25000000109246656 ) ) ;
#3597=CARTESIAN_POINT ( 'NONE',  ( 3.796994071234847710E-16, 61.93301269999999903, 44.95000000109246940 ) ) ;
#3605=CARTESIAN_POINT ( 'NONE',  ( -1.461580736456473906, 65.46158073645646880, 49.45000000109246940 ) ) ;
#3624=CARTESIAN_POINT ( 'NONE',  ( -1.035533905932738641, 66.50000000000000000, 49.15000000218494591 ) ) ;
#3625=DIRECTION ( 'NONE',  ( 1.000000000000000000, 1.734723475976807094E-15, -0.000000000000000000 ) ) ;
#3630=VERTEX_POINT ( 'NONE', #9435 ) ;
#3637=CARTESIAN_POINT ( 'NONE',  ( -2.066987300000001859, 64.85617417291294373, 48.70000000109247651 ) ) ;
#3638=VECTOR ( 'NONE', #15142, 1000.000000000000000 ) ;
#3639=CARTESIAN_POINT ( 'NONE',  ( -1.461580736456473906, 65.46158073645646880, 47.25000000109246656 ) ) ;
#3642=CARTESIAN_POINT ( 'NONE',  ( -1.530808498934192803E-16, 66.50000000000000000, 45.00000000000000000 ) ) ;
#3658=CARTESIAN_POINT ( 'NONE',  ( -1.530808498934192803E-16, 66.50000000000000000, 45.10000000218494165 ) ) ;
#3666=LINE ( 'NONE', #6616, #3950 ) ;
#3672=MECHANICAL_DESIGN_GEOMETRIC_PRESENTATION_REPRESENTATION('',(#5247),#6190);
#3675=DIRECTION ( 'NONE',  ( 0.000000000000000000, -0.000000000000000000, 1.000000000000000000 ) ) ;
#3684=CARTESIAN_POINT ( 'NONE',  ( 0.8561741729129472844, 61.93301270000000613, 47.60000000109246798 ) ) ;
#3698=CARTESIAN_POINT ( 'NONE',  ( -2.066987300000001415, 64.85617417291294373, 45.50000000109247367 ) ) ;
#3702=CARTESIAN_POINT ( 'NONE',  ( -7.999999999999986677, 68.00000000000000000, 66.99999999999997158 ) ) ;
#3705=ORIENTED_EDGE ( 'NONE', *, *, #10956, .T. ) ;
#3707=( LENGTH_UNIT ( ) NAMED_UNIT ( * ) SI_UNIT ( .MILLI., .METRE. ) );
#3715=CARTESIAN_POINT ( 'NONE',  ( 2.500000000000001776, 64.00000000000000000, 48.90000000218494591 ) ) ;
#3723=CARTESIAN_POINT ( 'NONE',  ( 0.5387381024323600887, 61.98586169951557423, 44.99999999999999289 ) ) ;
#3727=CARTESIAN_POINT ( 'NONE',  ( -1.461580736456473462, 62.53841926354353120, 47.25000000109247367 ) ) ;
#3728=CARTESIAN_POINT ( 'NONE',  ( -1.265664690411616068E-16, 66.06698730000000808, 48.75000000109246656 ) ) ;
#3729=CARTESIAN_POINT ( 'NONE',  ( -4.999999999999980460, 60.00000000000000711, 69.99999999999998579 ) ) ;
#3762=UNCERTAINTY_MEASURE_WITH_UNIT (LENGTH_MEASURE( 1.000000000000000082E-05 ), #3707, 'distance_accuracy_value', 'NONE');
#3774=CARTESIAN_POINT ( 'NONE',  ( 1.767766952966369987, 65.76776695296638309, 46.60000000218494165 ) ) ;
#3783=CARTESIAN_POINT ( 'NONE',  ( -0.8561741729129461742, 66.06698729999999387, 44.80000000109246372 ) ) ;
#3797=DIRECTION ( 'NONE',  ( -0.000000000000000000, -0.000000000000000000, -1.000000000000000000 ) ) ;
#3800=CARTESIAN_POINT ( 'NONE',  ( 2.066987300000001415, 64.00000000000000000, 45.15000000109247225 ) ) ;
#3802=CARTESIAN_POINT ( 'NONE',  ( -2.500000000000001776, 64.00000000000000000, 49.30000000218494449 ) ) ;
#3816=CARTESIAN_POINT ( 'NONE',  ( -1.035533905932738863, 61.50000000000000000, 46.25000000218494733 ) ) ;
#3817=DIRECTION ( 'NONE',  ( 0.000000000000000000, 0.000000000000000000, 1.000000000000000000 ) ) ;
#3823=CARTESIAN_POINT ( 'NONE',  ( -1.366300952416055425, 62.44303698707672368, 45.00000000000000711 ) ) ;
#3826=CARTESIAN_POINT ( 'NONE',  ( -0.8561741729129461742, 66.06698729999999387, 44.60000000109246088 ) ) ;
#3827=CARTESIAN_POINT ( 'NONE',  ( -0.8561741729129461742, 66.06698730000000808, 49.60000000109247509 ) ) ;
#3870=CARTESIAN_POINT ( 'NONE',  ( -1.265664690411616068E-16, 66.06698730000000808, 45.55000000109246372 ) ) ;
#3891=ADVANCED_FACE ( 'NONE', ( #7656 ), #13622, .T. ) ;
#3905=CARTESIAN_POINT ( 'NONE',  ( -1.767766952966370209, 65.76776695296638309, 49.20000000218494307 ) ) ;
#3906=LINE ( 'NONE', #8325, #8745 ) ;
#3911=ORIENTED_EDGE ( 'NONE', *, *, #5520, .F. ) ;
#3915=CARTESIAN_POINT ( 'NONE',  ( -0.8561741729129465073, 61.93301270000000613, 44.90000000109247225 ) ) ;
#3920=CARTESIAN_POINT ( 'NONE',  ( 2.154726813346381942, 63.29944981661203229, 45.00000000000002842 ) ) ;
#3950=VECTOR ( 'NONE', #12672, 1000.000000000000000 ) ;
#3958=MANIFOLD_SOLID_BREP ( 'Cavity1', #7554 ) ;
#3969=CARTESIAN_POINT ( 'NONE',  ( 1.767766952966369987, 65.76776695296638309, 49.69999999999999574 ) ) ;
#3977=CARTESIAN_POINT ( 'NONE',  ( -1.767766952966370209, 65.76776695296638309, 49.09999999999999432 ) ) ;
#3983=CARTESIAN_POINT ( 'NONE',  ( 0.8561741729129460632, 66.06698730000000808, 46.10000000109246798 ) ) ;
#4000=CARTESIAN_POINT ( 'NONE',  ( 2.500000000000002220, 62.96446609406726935, 47.25000000218494023 ) ) ;
#4010=CARTESIAN_POINT ( 'NONE',  ( -2.066987300000001415, 63.14382582708705627, 46.40000000109246514 ) ) ;
#4013=CARTESIAN_POINT ( 'NONE',  ( -2.500000000000003553, 62.96446609406726225, 49.24999999999997868 ) ) ;
#4032=AXIS2_PLACEMENT_3D ( 'NONE', #13057, #15738, #11490 ) ;
#4047=CARTESIAN_POINT ( 'NONE',  ( -1.035533905932738863, 61.50000000000000000, 48.54999999999999716 ) ) ;
#4062=CARTESIAN_POINT ( 'NONE',  ( -1.767766952966370209, 65.76776695296638309, 49.89999999999999147 ) ) ;
#4078=CARTESIAN_POINT ( 'NONE',  ( 2.066987300000001859, 63.14382582708704916, 46.70000000109248361 ) ) ;
#4096=ORIENTED_EDGE ( 'NONE', *, *, #6380, .T. ) ;
#4101=CARTESIAN_POINT ( 'NONE',  ( 2.066987300000002303, 63.14382582708705627, 48.30000000109247082 ) ) ;
#4114=CARTESIAN_POINT ( 'NONE',  ( -0.8561741729129461742, 66.06698729999999387, 49.60000000109246798 ) ) ;
#4122=VERTEX_POINT ( 'NONE', #11530 ) ;
#4124=( BOUNDED_SURFACE ( )  B_SPLINE_SURFACE ( 1, 2, ( 
 ( #9701, #12358, #8063, #9418, #14125, #12266, #11167, #6490, #2263, #6589, #3355, #12454, #6682, #4928, #4831, #15412, #7867, #3637, #1980, #16783, #700, #9320, #7963, #14217, #5022, #5124, #10980, #410, #13928, #10885, #16880, #16985, #12556, #6395, #3544, #18356, #14023, #595, #11077, #17075, #9609, #15595, #12647, #18645, #5212, #17166, #3727, #15693, #6296, #10072, #875, #14309, #9884, #1164, #17440, #15974, #7141, #6854, #9973, #2440, #1067, #18733, #11256, #4010, #4209, #8334, #6952, #19014, #5484, #2537, #12827, #8520, #976, #11447, #13109, #5298, #9793, #8423, #15786, #11538, #17258, #18824, #5579, #12737, #14494, #17347, #16066, #2626, #5398, #784, #17536, #19109, #11354, #3915, #7044, #15878, #14595, #16162, #6771, #3826, #13014 ),
 ( #2732, #10161, #11642, #4114, #2351, #5682, #14399, #8611, #17633, #18917, #8703, #12923, #16458, #5873, #10661, #16556, #14688, #9103, #8904, #2926, #4706, #12036, #11835, #7243, #15092, #1266, #10369, #16662, #7435, #13512, #14891, #16255, #17832, #13305, #19305, #4408, #14986, #14796, #16363, #13214, #3025, #4308, #13403, #2828, #1367, #9002, #19205, #1466, #7336, #10265, #4609, #8809, #14522, #10564, #5975, #11944, #17936, #1665, #4507, #10463, #7638, #1561, #7537, #92, #6072, #5774, #11734, #18032, #18129, #3123, #13605, #188, #6174, #12136, #3227, #17731, #9386, #5182, #18233, #4808, #6462, #10757, #3520, #15383, #6655, #385, #16756, #16956, #11141, #10860, #1953, #16854, #7740, #3415, #17138, #9296, #6559, #8033, #2139, #7938, #13998 ) ),
 .UNSPECIFIED., .F., .F., .F. ) 
 B_SPLINE_SURFACE_WITH_KNOTS ( ( 2, 2 ),
 ( 3, 2, 2, 2, 2, 2, 2, 2, 2, 2, 2, 2, 2, 2, 2, 2, 2, 2, 2, 2, 2, 2, 2, 2, 2, 2, 2, 2, 2, 2, 2, 2, 2, 2, 2, 2, 2, 2, 2, 2, 2, 2, 2, 2, 2, 2, 2, 2, 2, 2, 3 ),
 ( 0.000000000000000000, 1.000000000000000000 ),
 ( 0.000000000000000000, 0.01785714285714285615, 0.03571428571428571230, 0.05357142857142856845, 0.07142857142857142461, 0.08928571428571428770, 0.1071428571428571369, 0.1250000000000000000, 0.1428571428571428492, 0.1607142857142857262, 0.1785714285714285754, 0.1964285714285714246, 0.2142857142857142738, 0.2321428571428571508, 0.2500000000000000000, 0.2678571428571428492, 0.2857142857142856984, 0.3035714285714285476, 0.3214285714285714524, 0.3392857142857143016, 0.3571428571428571508, 0.3750000000000000000, 0.3928571428571428492, 0.4107142857142856984, 0.4285714285714285476, 0.4464285714285714524, 0.4642857142857143016, 0.4821428571428571508, 0.5000000000000000000, 0.5178571428571429047, 0.5357142857142856984, 0.5535714285714286031, 0.5714285714285713969, 0.5892857142857143016, 0.6071428571428570953, 0.6250000000000000000, 0.6428571428571429047, 0.6607142857142856984, 0.6785714285714286031, 0.6964285714285713969, 0.7142857142857143016, 0.7321428571428570953, 0.7500000000000000000, 0.7678571428571429047, 0.7857142857142856984, 0.8035714285714286031, 0.8214285714285713969, 0.8392857142857143016, 0.8571428571428570953, 0.8750000000000000000, 0.8928571428571429047 ),
 .UNSPECIFIED. ) 
 GEOMETRIC_REPRESENTATION_ITEM ( )  RATIONAL_B_SPLINE_SURFACE ( (
 ( 1.000000000000000000, 0.9238795325112867385, 1.000000000000000000, 0.9238795325112867385, 1.000000000000000000, 0.9238795325112867385, 1.000000000000000000, 0.9238795325112867385, 1.000000000000000000, 0.9238795325112867385, 1.000000000000000000, 0.9238795325112867385, 1.000000000000000000, 0.9238795325112867385, 1.000000000000000000, 0.9238795325112867385, 1.000000000000000000, 0.9238795325112867385, 1.000000000000000000, 0.9238795325112867385, 1.000000000000000000, 0.9238795325112867385, 1.000000000000000000, 0.9238795325112867385, 1.000000000000000000, 0.9238795325112867385, 1.000000000000000000, 0.9238795325112867385, 1.000000000000000000, 0.9238795325112867385, 1.000000000000000000, 0.9238795325112867385, 1.000000000000000000, 0.9238795325112867385, 1.000000000000000000, 0.9238795325112867385, 1.000000000000000000, 0.9238795325112867385, 1.000000000000000000, 0.9238795325112867385, 1.000000000000000000, 0.9238795325112867385, 1.000000000000000000, 0.9238795325112867385, 1.000000000000000000, 0.9238795325112867385, 1.000000000000000000, 0.9238795325112867385, 1.000000000000000000, 0.9238795325112867385, 1.000000000000000000, 0.9238795325112867385, 1.000000000000000000, 0.9238795325112867385, 1.000000000000000000, 0.9238795325112867385, 1.000000000000000000, 0.9238795325112867385, 1.000000000000000000, 0.9238795325112867385, 1.000000000000000000, 0.9238795325112867385, 1.000000000000000000, 0.9238795325112867385, 1.000000000000000000, 0.9238795325112867385, 1.000000000000000000, 0.9238795325112867385, 1.000000000000000000, 0.9238795325112867385, 1.000000000000000000, 0.9238795325112867385, 1.000000000000000000, 0.9238795325112867385, 1.000000000000000000, 0.9238795325112867385, 1.000000000000000000, 0.9238795325112867385, 1.000000000000000000, 0.9238795325112867385, 1.000000000000000000, 0.9238795325112867385, 1.000000000000000000, 0.9238795325112867385, 1.000000000000000000, 0.9238795325112867385, 1.000000000000000000, 0.9238795325112867385, 1.000000000000000000, 0.9238795325112867385, 1.000000000000000000, 0.9238795325112867385, 1.000000000000000000, 0.9238795325112867385, 1.000000000000000000, 0.9238795325112867385, 1.000000000000000000, 0.9238795325112867385, 1.000000000000000000, 0.9238795325112867385, 1.000000000000000000),
 ( 1.000000000000000000, 0.9238795325112867385, 1.000000000000000000, 0.9238795325112867385, 1.000000000000000000, 0.9238795325112867385, 1.000000000000000000, 0.9238795325112867385, 1.000000000000000000, 0.9238795325112867385, 1.000000000000000000, 0.9238795325112867385, 1.000000000000000000, 0.9238795325112867385, 1.000000000000000000, 0.9238795325112867385, 1.000000000000000000, 0.9238795325112867385, 1.000000000000000000, 0.9238795325112867385, 1.000000000000000000, 0.9238795325112867385, 1.000000000000000000, 0.9238795325112867385, 1.000000000000000000, 0.9238795325112867385, 1.000000000000000000, 0.9238795325112867385, 1.000000000000000000, 0.9238795325112867385, 1.000000000000000000, 0.9238795325112867385, 1.000000000000000000, 0.9238795325112867385, 1.000000000000000000, 0.9238795325112867385, 1.000000000000000000, 0.9238795325112867385, 1.000000000000000000, 0.9238795325112867385, 1.000000000000000000, 0.9238795325112867385, 1.000000000000000000, 0.9238795325112867385, 1.000000000000000000, 0.9238795325112867385, 1.000000000000000000, 0.9238795325112867385, 1.000000000000000000, 0.9238795325112867385, 1.000000000000000000, 0.9238795325112867385, 1.000000000000000000, 0.9238795325112867385, 1.000000000000000000, 0.9238795325112867385, 1.000000000000000000, 0.9238795325112867385, 1.000000000000000000, 0.9238795325112867385, 1.000000000000000000, 0.9238795325112867385, 1.000000000000000000, 0.9238795325112867385, 1.000000000000000000, 0.9238795325112867385, 1.000000000000000000, 0.9238795325112867385, 1.000000000000000000, 0.9238795325112867385, 1.000000000000000000, 0.9238795325112867385, 1.000000000000000000, 0.9238795325112867385, 1.000000000000000000, 0.9238795325112867385, 1.000000000000000000, 0.9238795325112867385, 1.000000000000000000, 0.9238795325112867385, 1.000000000000000000, 0.9238795325112867385, 1.000000000000000000, 0.9238795325112867385, 1.000000000000000000, 0.9238795325112867385, 1.000000000000000000, 0.9238795325112867385, 1.000000000000000000, 0.9238795325112867385, 1.000000000000000000, 0.9238795325112867385, 1.000000000000000000, 0.9238795325112867385, 1.000000000000000000, 0.9238795325112867385, 1.000000000000000000, 0.9238795325112867385, 1.000000000000000000, 0.9238795325112867385, 1.000000000000000000) ) ) 
 REPRESENTATION_ITEM ( '' )  SURFACE ( )  );
#4145=DIRECTION ( 'NONE',  ( 0.000000000000000000, -0.000000000000000000, -1.000000000000000000 ) ) ;
#4169=CARTESIAN_POINT ( 'NONE',  ( -1.461580736456473906, 65.46158073645646880, 45.65000000109247225 ) ) ;
#4176=CARTESIAN_POINT ( 'NONE',  ( -2.499999999999999112, 65.03553390593273775, 49.15000000000000568 ) ) ;
#4185=CARTESIAN_POINT ( 'NONE',  ( 1.461580736456473684, 65.46158073645646880, 49.45000000109246940 ) ) ;
#4192=CARTESIAN_POINT ( 'NONE',  ( -2.500000000000003997, 65.03553390593273775, 47.55000000000000426 ) ) ;
#4198=CARTESIAN_POINT ( 'NONE',  ( -2.066987300000001859, 64.85617417291294373, 48.70000000109247651 ) ) ;
#4209=CARTESIAN_POINT ( 'NONE',  ( -2.066987300000001415, 64.00000000000000000, 46.35000000109246798 ) ) ;
#4226=CARTESIAN_POINT ( 'NONE',  ( -7.999999999999986677, 60.00000000000000711, 45.00000000000000000 ) ) ;
#4227=ORIENTED_EDGE ( 'NONE', *, *, #16848, .T. ) ;
#4235=( BOUNDED_CURVE ( )  B_SPLINE_CURVE ( 2, ( #2183, #12666, #6792, #5417, #3658, #15612, #8267 ),
 .UNSPECIFIED., .F., .F. ) 
 B_SPLINE_CURVE_WITH_KNOTS ( ( 3, 2, 2, 3 ),
 ( 0.7142857142857141906, 0.7321428571428569843, 0.7500000000000000000, 0.7678571432794591978 ),
 .UNSPECIFIED. ) 
 CURVE ( )  GEOMETRIC_REPRESENTATION_ITEM ( )  RATIONAL_B_SPLINE_CURVE ( ( 1.000000000000000444, 0.9238795325112862944, 1.000000000000000000, 0.9238795325112867385, 1.000000000000000000, 0.9238795325112867385, 1.000000000000000000 ) ) 
 REPRESENTATION_ITEM ( '' )  );
#4251=ORIENTED_EDGE ( 'NONE', *, *, #2645, .F. ) ;
#4265=CARTESIAN_POINT ( 'NONE',  ( -1.530808498934192803E-16, 66.50000000000000000, 45.79999999999999005 ) ) ;
#4279=EDGE_CURVE ( 'NONE', #663, #7431, #14249, .T. ) ;
#4282=CYLINDRICAL_SURFACE ( 'NONE', #16332, 2.500000000000001776 ) ;
#4283=CARTESIAN_POINT ( 'NONE',  ( 2.066987300000001415, 64.85617417291294373, 48.60000000109246798 ) ) ;
#4298=CARTESIAN_POINT ( 'NONE',  ( -1.530808498934192803E-16, 66.50000000000000000, 45.90000000218494591 ) ) ;
#4304=DIRECTION ( 'NONE',  ( 0.000000000000000000, -1.000000000000000000, 0.000000000000000000 ) ) ;
#4308=CARTESIAN_POINT ( 'NONE',  ( 2.066987300000002303, 63.14382582708705627, 47.70000000109247651 ) ) ;
#4348=ORIENTED_EDGE ( 'NONE', *, *, #3519, .F. ) ;
#4362=CARTESIAN_POINT ( 'NONE',  ( 1.035533905932739751, 61.50000000000000000, 47.85000000000000142 ) ) ;
#4379=ADVANCED_FACE ( 'NONE', ( #4600 ), #10558, .F. ) ;
#4391=CARTESIAN_POINT ( 'NONE',  ( 1.767766952966369987, 65.76776695296638309, 47.29999999999999716 ) ) ;
#4398=CARTESIAN_POINT ( 'NONE',  ( 1.035533905932738197, 66.50000000000000000, 48.14999999999999858 ) ) ;
#4399=CARTESIAN_POINT ( 'NONE',  ( 1.461580736456473906, 62.53841926354353120, 49.05000000109247082 ) ) ;
#4407=AXIS2_PLACEMENT_3D ( 'NONE', #10565, #4409, #17937 ) ;
#4408=CARTESIAN_POINT ( 'NONE',  ( -0.8561741729129461742, 66.06698729999999387, 48.00000000109246656 ) ) ;
#4409=DIRECTION ( 'NONE',  ( 0.000000000000000000, 0.000000000000000000, -1.000000000000000000 ) ) ;
#4446=AXIS2_PLACEMENT_3D ( 'NONE', #2564, #7273, #4145 ) ;
#4447=CARTESIAN_POINT ( 'NONE',  ( 1.035533905932739751, 61.50000000000000000, 47.95000000218494307 ) ) ;
#4451=AXIS2_PLACEMENT_3D ( 'NONE', #7178, #14630, #1194 ) ;
#4465=CARTESIAN_POINT ( 'NONE',  ( 2.500000000000001776, 65.03553390593273775, 48.04999999999999716 ) ) ;
#4472=CARTESIAN_POINT ( 'NONE',  ( -1.218482738863178705, 66.05435652614266928, 44.99999999999999289 ) ) ;
#4482=FACE_OUTER_BOUND ( 'NONE', #7490, .T. ) ;
#4483=CARTESIAN_POINT ( 'NONE',  ( -1.461580736456473462, 62.53841926354353120, 45.85000000109246798 ) ) ;
#4496=CARTESIAN_POINT ( 'NONE',  ( 4.592425496802577917E-16, 61.50000000000000000, 48.70000000218494307 ) ) ;
#4499=CARTESIAN_POINT ( 'NONE',  ( -1.530808498934192803E-16, 66.50000000000000000, 45.10000000218494165 ) ) ;
#4507=CARTESIAN_POINT ( 'NONE',  ( 1.461580736456473906, 62.53841926354353120, 46.85000000109246798 ) ) ;
#4509=EDGE_CURVE ( 'NONE', #14847, #14201, #6977, .T. ) ;
#4522=CARTESIAN_POINT ( 'NONE',  ( 4.592425496802577917E-16, 61.50000000000000000, 47.10000000218494165 ) ) ;
#4559=CARTESIAN_POINT ( 'NONE',  ( -1.767766952966370209, 65.76776695296638309, 45.89999999999999858 ) ) ;
#4572=LINE ( 'NONE', #7906, #10476 ) ;
#4580=CARTESIAN_POINT ( 'NONE',  ( 1.461580736456473684, 65.46158073645646880, 45.45000000109246940 ) ) ;
#4597=CARTESIAN_POINT ( 'NONE',  ( 2.066987300000002303, 63.14382582708705627, 47.50000000109246656 ) ) ;
#4600=FACE_OUTER_BOUND ( 'NONE', #14380, .T. ) ;
#4609=CARTESIAN_POINT ( 'NONE',  ( -1.461580736456473906, 65.46158073645646880, 47.25000000109246656 ) ) ;
#4636=B_SPLINE_CURVE_WITH_KNOTS ( 'NONE', 3,
 ( #1526, #17900, #16217, #16418, #1330, #19268, #19363, #15051, #7400, #13471, #5931, #12094, #4472, #245, #7599, #13371, #2983, #8963 ),
 .UNSPECIFIED., .F., .F.,
 ( 4, 2, 2, 2, 2, 2, 2, 2, 4 ),
 ( 0.000000000000000000, 0.0005608035642034970908, 0.001121607128406994182, 0.001682410692610491381, 0.002243214256813988363, 0.002804017821017484695, 0.003364821385220981894, 0.003925624949424478226, 0.004486428513627974991 ),
 .UNSPECIFIED. ) ;
#4638=CARTESIAN_POINT ( 'NONE',  ( -1.767766952966369765, 62.23223304703363112, 46.20000000218494307 ) ) ;
#4651=ORIENTED_EDGE ( 'NONE', *, *, #13942, .T. ) ;
#4657=CARTESIAN_POINT ( 'NONE',  ( 0.000000000000000000, 64.00000000000000000, 49.99999999999999289 ) ) ;
#4680=CYLINDRICAL_SURFACE ( 'NONE', #16476, 2.500000000000001776 ) ;
#4693=CARTESIAN_POINT ( 'NONE',  ( -1.035533905932738641, 66.50000000000000000, 48.24999999999999289 ) ) ;
#4694=CARTESIAN_POINT ( 'NONE',  ( 2.066987300000001859, 64.85617417291294373, 47.60000000109246798 ) ) ;
#4698=EDGE_CURVE ( 'NONE', #10838, #18337, #17227, .T. ) ;
#4702=CARTESIAN_POINT ( 'NONE',  ( 1.461580736456473684, 65.46158073645646880, 49.25000000109246656 ) ) ;
#4706=CARTESIAN_POINT ( 'NONE',  ( -1.265664690411616068E-16, 66.06698730000000808, 48.75000000109246656 ) ) ;
#4710=CARTESIAN_POINT ( 'NONE',  ( 2.500000000000001776, 64.00000000000000000, 45.70000000218494307 ) ) ;
#4711=ORIENTED_EDGE ( 'NONE', *, *, #14177, .F. ) ;
#4728=CARTESIAN_POINT ( 'NONE',  ( 4.592425496802577917E-16, 61.50000000000000000, 45.39999999999999858 ) ) ;
#4755=AXIS2_PLACEMENT_3D ( 'NONE', #13630, #2951, #10491 ) ;
#4783=LINE ( 'NONE', #16227, #581 ) ;
#4787=CARTESIAN_POINT ( 'NONE',  ( 2.066987300000001415, 64.85617417291294373, 46.20000000109248361 ) ) ;
#4788=CARTESIAN_POINT ( 'NONE',  ( 2.066987300000002303, 63.14382582708705627, 49.30000000109246372 ) ) ;
#4800=CARTESIAN_POINT ( 'NONE',  ( -0.8561741729129461742, 66.06698729999999387, 45.40000000109246514 ) ) ;
#4806=CARTESIAN_POINT ( 'NONE',  ( -0.8561741729129466183, 61.93301270000000613, 48.10000000109246798 ) ) ;
#4808=CARTESIAN_POINT ( 'NONE',  ( -2.066987300000001415, 63.14382582708705627, 45.80000000109246372 ) ) ;
#4815=DIRECTION ( 'NONE',  ( 0.000000000000000000, 0.000000000000000000, 1.000000000000000000 ) ) ;
#4825=CARTESIAN_POINT ( 'NONE',  ( 1.035533905932739751, 61.50000000000000000, 45.44999999999999574 ) ) ;
#4831=CARTESIAN_POINT ( 'NONE',  ( -1.461580736456473462, 62.53841926354353120, 48.85000000109246798 ) ) ;
#4866=CARTESIAN_POINT ( 'NONE',  ( 2.500000000000001776, 64.00000000000000000, 48.10000000218494165 ) ) ;
#4874=CARTESIAN_POINT ( 'NONE',  ( 0.000000000000000000, 64.00000000000000000, 49.99999999999999289 ) ) ;
#4876=CARTESIAN_POINT ( 'NONE',  ( 0.8561741729129472844, 61.93301270000000613, 46.80000000109246372 ) ) ;
#4879=ORIENTED_EDGE ( 'NONE', *, *, #6769, .T. ) ;
#4883=EDGE_LOOP ( 'NONE', ( #1540, #2610, #3452, #10657 ) ) ;
#4890=CARTESIAN_POINT ( 'NONE',  ( 2.066987300000002303, 63.14382582708705627, 45.10000000109246798 ) ) ;
#4892=EDGE_CURVE ( 'NONE', #6563, #9100, #14539, .T. ) ;
#4897=CARTESIAN_POINT ( 'NONE',  ( 1.461580736456473906, 62.53841926354353120, 49.05000000109247082 ) ) ;
#4904=CARTESIAN_POINT ( 'NONE',  ( 1.767766952966370653, 62.23223304703363112, 45.60000000218494165 ) ) ;
#4923=ORIENTED_EDGE ( 'NONE', *, *, #4509, .F. ) ;
#4928=CARTESIAN_POINT ( 'NONE',  ( -0.8561741729129465073, 61.93301270000000613, 48.90000000109247225 ) ) ;
#4933=CARTESIAN_POINT ( 'NONE',  ( -2.066987300000001415, 64.00000000000000000, 49.75000000109246656 ) ) ;
#4946=CARTESIAN_POINT ( 'NONE',  ( -2.066987300000001415, 64.00000000000000000, 49.65000000109247225 ) ) ;
#4971=CARTESIAN_POINT ( 'NONE',  ( -1.767766952966370209, 65.76776695296638309, 48.40000000218494591 ) ) ;
#4972=CARTESIAN_POINT ( 'NONE',  ( 1.461580736456473684, 65.46158073645646880, 48.65000000109247225 ) ) ;
#4986=CARTESIAN_POINT ( 'NONE',  ( 0.8561741729129472844, 61.93301270000000613, 45.00000000109246656 ) ) ;
#4993=CARTESIAN_POINT ( 'NONE',  ( -1.265664690411616068E-16, 66.06698730000000808, 49.35000000109246798 ) ) ;
#4995=DIRECTION ( 'NONE',  ( 0.000000000000000000, 0.000000000000000000, 1.000000000000000000 ) ) ;
#5022=CARTESIAN_POINT ( 'NONE',  ( 2.066987300000001415, 64.00000000000000000, 48.35000000109246798 ) ) ;
#5028=EDGE_LOOP ( 'NONE', ( #6303, #9952, #16859, #4251 ) ) ;
#5043=VECTOR ( 'NONE', #13923, 1000.000000000000000 ) ;
#5053=AXIS2_PLACEMENT_3D ( 'NONE', #11050, #17047, #9200 ) ;
#5072=CARTESIAN_POINT ( 'NONE',  ( -0.8561741729129465073, 61.93301270000000613, 49.10000000109246088 ) ) ;
#5086=CARTESIAN_POINT ( 'NONE',  ( 1.767766952966370653, 62.23223304703363112, 48.69999999999999574 ) ) ;
#5093=DIRECTION ( 'NONE',  ( -0.000000000000000000, -0.000000000000000000, -1.000000000000000000 ) ) ;
#5094=CYLINDRICAL_SURFACE ( 'NONE', #5053, 2.500000000000001776 ) ;
#5104=VERTEX_POINT ( 'NONE', #8248 ) ;
#5124=CARTESIAN_POINT ( 'NONE',  ( 2.066987300000002303, 63.14382582708705627, 48.30000000109247082 ) ) ;
#5126=CARTESIAN_POINT ( 'NONE',  ( 3.796994071234847710E-16, 61.93301269999999903, 49.15000000109246514 ) ) ;
#5129=CARTESIAN_POINT ( 'NONE',  ( 2.227674122569385240, 64.95406575718618569, 45.00000000000000711 ) ) ;
#5155=CARTESIAN_POINT ( 'NONE',  ( -2.500000000000001776, 62.96446609406726225, 46.84999999999998721 ) ) ;
#5161=CARTESIAN_POINT ( 'NONE',  ( 2.066987300000001415, 64.00000000000000000, 48.55000000109247082 ) ) ;
#5178=CARTESIAN_POINT ( 'NONE',  ( 1.461580736456473684, 65.46158073645646880, 46.05000000109246372 ) ) ;
#5182=CARTESIAN_POINT ( 'NONE',  ( -0.8561741729129465073, 61.93301270000000613, 45.90000000109247225 ) ) ;
#5184=CARTESIAN_POINT ( 'NONE',  ( 2.500000000000001776, 64.00000000000000000, 47.30000000218494449 ) ) ;
#5185=ORIENTED_EDGE ( 'NONE', *, *, #2293, .T. ) ;
#5193=ORIENTED_EDGE ( 'NONE', *, *, #6915, .F. ) ;
#5198=CARTESIAN_POINT ( 'NONE',  ( 4.592425496802577917E-16, 61.50000000000000000, 47.90000000218494591 ) ) ;
#5212=CARTESIAN_POINT ( 'NONE',  ( 3.796994071234847710E-16, 61.93301269999999903, 47.35000000109246798 ) ) ;
#5214=CARTESIAN_POINT ( 'NONE',  ( 3.796994071234847710E-16, 61.93301269999999903, 46.75000000109246656 ) ) ;
#5224=VECTOR ( 'NONE', #15223, 1000.000000000000000 ) ;
#5247=STYLED_ITEM ( 'NONE', ( #14778 ), #12018 ) ;
#5257=CARTESIAN_POINT ( 'NONE',  ( 3.796994071234847710E-16, 61.93301269999999903, 45.95000000109246940 ) ) ;
#5266=( BOUNDED_CURVE ( )  B_SPLINE_CURVE ( 2, ( #740, #14074, #4971, #15551, #1828, #6346, #3302, #10835, #9271 ),
 .UNSPECIFIED., .F., .F. ) 
 B_SPLINE_CURVE_WITH_KNOTS ( ( 3, 2, 2, 2, 3 ),
 ( 0.1428571428571428215, 0.1607142857142856429, 0.1785714285714284644, 0.1964285714285712858, 0.2142857142857140795 ),
 .UNSPECIFIED. ) 
 CURVE ( )  GEOMETRIC_REPRESENTATION_ITEM ( )  RATIONAL_B_SPLINE_CURVE ( ( 1.000000000000000222, 0.9238795325112866275, 1.000000000000000000, 0.9238795325112867385, 1.000000000000000000, 0.9238795325112867385, 1.000000000000000000, 0.9238795325112875156, 0.9999999999999992228 ) ) 
 REPRESENTATION_ITEM ( '' )  );
#5269=CARTESIAN_POINT ( 'NONE',  ( 1.461580736456473906, 62.53841926354353120, 45.05000000109246372 ) ) ;
#5284=CARTESIAN_POINT ( 'NONE',  ( 1.767766952966369987, 65.76776695296638309, 47.40000000218494591 ) ) ;
#5298=CARTESIAN_POINT ( 'NONE',  ( 0.8561741729129472844, 61.93301270000000613, 45.80000000109246372 ) ) ;
#5299=CARTESIAN_POINT ( 'NONE',  ( 0.8561741729129471734, 61.93301270000000613, 49.20000000109247651 ) ) ;
#5302=CYLINDRICAL_SURFACE ( 'NONE', #11775, 2.500000000000001776 ) ;
#5348=CARTESIAN_POINT ( 'NONE',  ( 0.000000000000000000, 64.00000000000000000, 49.99999999999999289 ) ) ;
#5351=CARTESIAN_POINT ( 'NONE',  ( 0.8561741729129472844, 61.93301270000000613, 45.20000000109248361 ) ) ;
#5355=ORIENTED_EDGE ( 'NONE', *, *, #4279, .T. ) ;
#5369=CARTESIAN_POINT ( 'NONE',  ( 2.066987300000001859, 63.14382582708704916, 45.10000000109246798 ) ) ;
#5377=EDGE_LOOP ( 'NONE', ( #5906, #19115, #6837, #14115, #5185, #14018 ) ) ;
#5379=VECTOR ( 'NONE', #2995, 1000.000000000000000 ) ;
#5387=CARTESIAN_POINT ( 'NONE',  ( -1.530808498934192803E-16, 66.50000000000000000, 48.30000000218494449 ) ) ;
#5398=CARTESIAN_POINT ( 'NONE',  ( 2.066987300000001415, 64.00000000000000000, 45.15000000109247225 ) ) ;
#5402=CARTESIAN_POINT ( 'NONE',  ( 2.336416577439934805, 64.02633867252365008, 44.99999999999999289 ) ) ;
#5417=CARTESIAN_POINT ( 'NONE',  ( -1.035533905932738641, 66.50000000000000000, 45.15000000218493881 ) ) ;
#5430=CARTESIAN_POINT ( 'NONE',  ( 2.500000000000007994, 62.96446609406726225, 48.74999999999999289 ) ) ;
#5432=ADVANCED_FACE ( 'NONE', ( #1754 ), #9484, .T. ) ;
#5444=CARTESIAN_POINT ( 'NONE',  ( -2.500000000000001776, 64.00000000000000000, 49.99999999999999289 ) ) ;
#5456=CARTESIAN_POINT ( 'NONE',  ( -0.8561741729129461742, 66.06698730000000808, 46.20000000109248361 ) ) ;
#5464=ORIENTED_EDGE ( 'NONE', *, *, #7592, .F. ) ;
#5473=CARTESIAN_POINT ( 'NONE',  ( -1.767766952966370209, 65.76776695296638309, 46.80000000218494449 ) ) ;
#5484=CARTESIAN_POINT ( 'NONE',  ( -1.265664690411616068E-16, 66.06698730000000808, 46.15000000109247225 ) ) ;
#5487=CARTESIAN_POINT ( 'NONE',  ( -2.500000000000001776, 64.00000000000000000, 46.10000000218494165 ) ) ;
#5501=VERTEX_POINT ( 'NONE', #7835 ) ;
#5507=PLANE ( 'NONE',  #4446 ) ;
#5520=EDGE_CURVE ( 'NONE', #17001, #14616, #12974, .T. ) ;
#5538=CARTESIAN_POINT ( 'NONE',  ( -1.461580736456473462, 62.53841926354353120, 45.05000000109246372 ) ) ;
#5552=CARTESIAN_POINT ( 'NONE',  ( 0.8561741729129471734, 61.93301270000000613, 47.40000000109247225 ) ) ;
#5555=DIRECTION ( 'NONE',  ( 1.734723475976807094E-15, -1.000000000000000000, 0.000000000000000000 ) ) ;
#5569=CARTESIAN_POINT ( 'NONE',  ( 3.796994071234847710E-16, 61.93301269999999903, 48.95000000109246940 ) ) ;
#5576=CARTESIAN_POINT ( 'NONE',  ( -0.2730872843520700810, 61.94666219239776694, 45.00000000000001421 ) ) ;
#5579=CARTESIAN_POINT ( 'NONE',  ( -1.461580736456473906, 65.46158073645646880, 45.45000000109246940 ) ) ;
#5582=CARTESIAN_POINT ( 'NONE',  ( -2.500000000000001776, 64.00000000000000000, 49.19999999999999574 ) ) ;
#5605=SHAPE_DEFINITION_REPRESENTATION ( #8792, #15288 ) ;
#5607=( BOUNDED_CURVE ( )  B_SPLINE_CURVE ( 2, ( #18203, #2014, #11021, #15544, #15347, #8003, #2114, #5155, #17113 ),
 .UNSPECIFIED., .F., .F. ) 
 B_SPLINE_CURVE_WITH_KNOTS ( ( 3, 2, 2, 2, 3 ),
 ( 0.5000000000000001110, 0.5178571428571430157, 0.5357142857142858094, 0.5535714285714286031, 0.5714285714285713969 ),
 .UNSPECIFIED. ) 
 CURVE ( )  GEOMETRIC_REPRESENTATION_ITEM ( )  RATIONAL_B_SPLINE_CURVE ( ( 0.9999999999999995559, 0.9238795325112871826, 1.000000000000000000, 0.9238795325112867385, 1.000000000000000000, 0.9238795325112867385, 1.000000000000000000, 0.9238795325112867385, 1.000000000000000000 ) ) 
 REPRESENTATION_ITEM ( '' )  );
#5624=PLANE ( 'NONE',  #14239 ) ;
#5633=CARTESIAN_POINT ( 'NONE',  ( 0.8561741729129460632, 66.06698729999999387, 45.50000000109247367 ) ) ;
#5652=CARTESIAN_POINT ( 'NONE',  ( -2.066987300000001415, 64.85617417291294373, 47.30000000109247082 ) ) ;
#5656=CARTESIAN_POINT ( 'NONE',  ( 0.000000000000000000, 64.00000000000000000, 45.00000000000000000 ) ) ;
#5668=CARTESIAN_POINT ( 'NONE',  ( 2.500000000000001776, 64.00000000000000000, 45.70000000218494307 ) ) ;
#5672=CARTESIAN_POINT ( 'NONE',  ( 1.035533905932739751, 61.50000000000000000, 46.24999999999999289 ) ) ;
#5682=CARTESIAN_POINT ( 'NONE',  ( 0.8561741729129460632, 66.06698729999999387, 49.50000000109246656 ) ) ;
#5700=VERTEX_POINT ( 'NONE', #14319 ) ;
#5722=CARTESIAN_POINT ( 'NONE',  ( 1.035533905932739751, 61.50000000000000000, 48.64999999999999858 ) ) ;
#5734=CARTESIAN_POINT ( 'NONE',  ( 1.035533905932739751, 61.50000000000000000, 45.45000000000000995 ) ) ;
#5749=CARTESIAN_POINT ( 'NONE',  ( -1.461580736456473462, 62.53841926354353120, 47.45000000109246230 ) ) ;
#5762=CARTESIAN_POINT ( 'NONE',  ( -1.265664690411616068E-16, 66.06698730000000808, 49.35000000109246798 ) ) ;
#5774=CARTESIAN_POINT ( 'NONE',  ( -2.066987300000001859, 64.85617417291294373, 46.50000000109246656 ) ) ;
#5796=ORIENTED_EDGE ( 'NONE', *, *, #16365, .T. ) ;
#5832=CARTESIAN_POINT ( 'NONE',  ( 2.500000000000001776, 65.03553390593273775, 47.24999999999999289 ) ) ;
#5858=CARTESIAN_POINT ( 'NONE',  ( 2.500000000000001776, 64.00000000000000000, 47.19999999999999574 ) ) ;
#5865=CARTESIAN_POINT ( 'NONE',  ( -2.500000000000001776, 64.00000000000000000, 45.30000000218493739 ) ) ;
#5867=ORIENTED_EDGE ( 'NONE', *, *, #6958, .F. ) ;
#5873=CARTESIAN_POINT ( 'NONE',  ( -0.8561741729129465073, 61.93301270000000613, 49.10000000109246088 ) ) ;
#5882=CARTESIAN_POINT ( 'NONE',  ( -1.530808498934192803E-16, 66.50000000000000000, 45.00000000000000000 ) ) ;
#5906=ORIENTED_EDGE ( 'NONE', *, *, #15756, .F. ) ;
#5909=CARTESIAN_POINT ( 'NONE',  ( 2.500000000000001776, 64.00000000000000000, 48.10000000218494165 ) ) ;
#5924=AXIS2_PLACEMENT_3D ( 'NONE', #15186, #16754, #16953 ) ;
#5926=CARTESIAN_POINT ( 'NONE',  ( -1.035533905932738863, 61.50000000000000000, 47.74999999999999289 ) ) ;
#5931=CARTESIAN_POINT ( 'NONE',  ( -1.633339126078534154, 65.67088701091057601, 44.99999999999999289 ) ) ;
#5947=CARTESIAN_POINT ( 'NONE',  ( -2.066987300000000971, 63.14382582708704916, 45.80000000109246372 ) ) ;
#5964=CARTESIAN_POINT ( 'NONE',  ( 1.767766952966370653, 62.23223304703363112, 44.80000000218493739 ) ) ;
#5968=CARTESIAN_POINT ( 'NONE',  ( 2.500000000000001776, 64.00000000000000000, 46.39999999999999858 ) ) ;
#5975=CARTESIAN_POINT ( 'NONE',  ( 1.461580736456473684, 65.46158073645646880, 47.05000000109247082 ) ) ;
#5980=ORIENTED_EDGE ( 'NONE', *, *, #4698, .T. ) ;
#5986=ORIENTED_EDGE ( 'NONE', *, *, #3297, .T. ) ;
#5991=CARTESIAN_POINT ( 'NONE',  ( 1.035533905932739751, 61.50000000000000000, 47.15000000218494591 ) ) ;
#6015=CARTESIAN_POINT ( 'NONE',  ( -2.500000000000011102, 62.96446609406727646, 47.75000000218493312 ) ) ;
#6030=CARTESIAN_POINT ( 'NONE',  ( -2.500000000000000888, 62.96446609406726935, 46.04999999999999005 ) ) ;
#6049=CARTESIAN_POINT ( 'NONE',  ( 1.461580736456473684, 65.46158073645646880, 46.25000000109246656 ) ) ;
#6056=CARTESIAN_POINT ( 'NONE',  ( -1.767766952966370209, 65.76776695296638309, 47.49999999999999289 ) ) ;
#6062=LINE ( 'NONE', #3317, #6344 ) ;
#6063=CARTESIAN_POINT ( 'NONE',  ( -1.461580736456473462, 62.53841926354353120, 47.25000000109247367 ) ) ;
#6065=EDGE_LOOP ( 'NONE', ( #15366, #2806, #17176, #4348, #10583, #77, #16992, #5867, #17595, #16976, #12350, #1961, #1935, #3020, #10520, #5796 ) ) ;
#6067=CARTESIAN_POINT ( 'NONE',  ( -2.500000000000001776, 64.00000000000000000, 46.00000000000000000 ) ) ;
#6069=ORIENTED_EDGE ( 'NONE', *, *, #2927, .T. ) ;
#6072=CARTESIAN_POINT ( 'NONE',  ( -2.066987300000001415, 64.00000000000000000, 46.55000000109247082 ) ) ;
#6074=FACE_BOUND ( 'NONE', #9981, .T. ) ;
#6089=ORIENTED_EDGE ( 'NONE', *, *, #847, .T. ) ;
#6106=ORIENTED_EDGE ( 'NONE', *, *, #7816, .F. ) ;
#6114=AXIS2_PLACEMENT_3D ( 'NONE', #14044, #8081, #335 ) ;
#6121=CARTESIAN_POINT ( 'NONE',  ( 2.500000000000002220, 62.96446609406726935, 47.14999999999999858 ) ) ;
#6128=( BOUNDED_CURVE ( )  B_SPLINE_CURVE ( 2, ( #3802, #9944, #11227, #12897, #15943, #12986, #14369, #6927, #7018 ),
 .UNSPECIFIED., .F., .F. ) 
 B_SPLINE_CURVE_WITH_KNOTS ( ( 3, 2, 2, 2, 3 ),
 ( 0.000000000000000000, 0.01785714285714289085, 0.03571428571428578169, 0.05357142857142867254, 0.07142857142857156338 ),
 .UNSPECIFIED. ) 
 CURVE ( )  GEOMETRIC_REPRESENTATION_ITEM ( )  RATIONAL_B_SPLINE_CURVE ( ( 1.000000000000000000, 0.9238795325112867385, 1.000000000000000000, 0.9238795325112867385, 1.000000000000000000, 0.9238795325112867385, 1.000000000000000000, 0.9238795325112861834, 1.000000000000000666 ) ) 
 REPRESENTATION_ITEM ( '' )  );
#6147=CARTESIAN_POINT ( 'NONE',  ( 3.796994071234847710E-16, 61.93301269999999903, 45.15000000109247225 ) ) ;
#6148=CARTESIAN_POINT ( 'NONE',  ( -1.265664690411616068E-16, 66.06698730000000808, 49.55000000109247082 ) ) ;
#6165=CARTESIAN_POINT ( 'NONE',  ( -1.265664690411616068E-16, 66.06698730000000808, 47.75000000109246656 ) ) ;
#6174=CARTESIAN_POINT ( 'NONE',  ( 2.066987300000001415, 64.00000000000000000, 46.15000000109247225 ) ) ;
#6183=ORIENTED_EDGE ( 'NONE', *, *, #17872, .F. ) ;
#6190=( GEOMETRIC_REPRESENTATION_CONTEXT ( 3 ) GLOBAL_UNCERTAINTY_ASSIGNED_CONTEXT ( ( #7693 ) ) GLOBAL_UNIT_ASSIGNED_CONTEXT ( ( #8983, #11717, #14970 ) ) REPRESENTATION_CONTEXT ( 'NONE', 'WORKASPACE' ) );
#6197=CARTESIAN_POINT ( 'NONE',  ( 2.500000000000002220, 62.96446609406726225, 45.54999999999999005 ) ) ;
#6237=FACE_OUTER_BOUND ( 'NONE', #5377, .T. ) ;
#6243=CARTESIAN_POINT ( 'NONE',  ( 2.066987300000001859, 64.85617417291294373, 48.60000000109246798 ) ) ;
#6257=CARTESIAN_POINT ( 'NONE',  ( 2.500000000000001776, 64.00000000000000000, 47.99999999999999289 ) ) ;
#6258=CARTESIAN_POINT ( 'NONE',  ( -2.066987300000001415, 64.00000000000000000, 45.55000000109246372 ) ) ;
#6264=CARTESIAN_POINT ( 'NONE',  ( 2.066987300000001415, 64.00000000000000000, 49.15000000109247225 ) ) ;
#6290=CARTESIAN_POINT ( 'NONE',  ( 1.767766952966370653, 62.23223304703363112, 45.50000000000000000 ) ) ;
#6296=CARTESIAN_POINT ( 'NONE',  ( -2.066987300000001415, 64.00000000000000000, 47.15000000109247225 ) ) ;
#6303=ORIENTED_EDGE ( 'NONE', *, *, #17489, .F. ) ;
#6307=ORIENTED_EDGE ( 'NONE', *, *, #10956, .F. ) ;
#6310=AXIS2_PLACEMENT_3D ( 'NONE', #4226, #2847, #17855 ) ;
#6317=DIRECTION ( 'NONE',  ( 0.000000000000000000, 0.000000000000000000, 1.000000000000000000 ) ) ;
#6344=VECTOR ( 'NONE', #179, 1000.000000000000000 ) ;
#6346=CARTESIAN_POINT ( 'NONE',  ( 1.035533905932738197, 66.50000000000000000, 48.25000000218494733 ) ) ;
#6347=CARTESIAN_POINT ( 'NONE',  ( 0.8561741729129460632, 66.06698729999999387, 46.30000000109247082 ) ) ;
#6361=CARTESIAN_POINT ( 'NONE',  ( -2.066987300000001415, 63.14382582708705627, 46.40000000109246514 ) ) ;
#6369=CARTESIAN_POINT ( 'NONE',  ( -7.999999999999986677, 68.00000000000000000, 45.00000000000000000 ) ) ;
#6373=ORIENTED_EDGE ( 'NONE', *, *, #9822, .T. ) ;
#6380=EDGE_CURVE ( 'NONE', #9572, #6563, #334, .T. ) ;
#6386=EDGE_CURVE ( 'NONE', #17001, #17276, #429, .T. ) ;
#6388=CARTESIAN_POINT ( 'NONE',  ( -2.500000000000001776, 64.00000000000000000, 45.19999999999999574 ) ) ;
#6395=CARTESIAN_POINT ( 'NONE',  ( -2.066987300000001859, 64.85617417291294373, 47.90000000109247225 ) ) ;
#6400=CARTESIAN_POINT ( 'NONE',  ( 1.890020143386967000, 65.62319932110614218, 45.00000000000000711 ) ) ;
#6405=VERTEX_POINT ( 'NONE', #14043 ) ;
#6426=AXIS2_PLACEMENT_3D ( 'NONE', #8096, #17110, #3675 ) ;
#6441=CARTESIAN_POINT ( 'NONE',  ( 2.066987300000001415, 64.00000000000000000, 47.75000000109246656 ) ) ;
#6455=CARTESIAN_POINT ( 'NONE',  ( -1.461580736456473906, 65.46158073645646880, 47.05000000109247082 ) ) ;
#6458=CARTESIAN_POINT ( 'NONE',  ( 0.000000000000000000, 64.00000000000000000, 49.99999999999999289 ) ) ;
#6460=CARTESIAN_POINT ( 'NONE',  ( -2.066987300000001415, 64.00000000000000000, 49.55000000109247082 ) ) ;
#6462=CARTESIAN_POINT ( 'NONE',  ( -2.066987300000001415, 64.00000000000000000, 45.75000000109247367 ) ) ;
#6490=CARTESIAN_POINT ( 'NONE',  ( 2.066987300000001859, 64.85617417291294373, 49.20000000109247651 ) ) ;
#6504=EDGE_CURVE ( 'NONE', #11173, #1259, #4235, .T. ) ;
#6536=CARTESIAN_POINT ( 'NONE',  ( 1.461580736456473684, 65.46158073645646880, 47.05000000109247082 ) ) ;
#6555=DIRECTION ( 'NONE',  ( -0.000000000000000000, -0.000000000000000000, -1.000000000000000000 ) ) ;
#6557=CARTESIAN_POINT ( 'NONE',  ( -1.461580736456473906, 65.46158073645646880, 47.85000000109246798 ) ) ;
#6559=CARTESIAN_POINT ( 'NONE',  ( -2.066987300000001415, 64.00000000000000000, 44.95000000109246940 ) ) ;
#6563=VERTEX_POINT ( 'NONE', #9811 ) ;
#6580=FILL_AREA_STYLE ('',( #15588 ) ) ;
#6589=CARTESIAN_POINT ( 'NONE',  ( 2.066987300000002303, 63.14382582708705627, 49.10000000109246088 ) ) ;
#6590=CARTESIAN_POINT ( 'NONE',  ( 2.066987300000001859, 63.14382582708704916, 46.90000000109247225 ) ) ;
#6615=PLANE ( 'NONE',  #18526 ) ;
#6616=CARTESIAN_POINT ( 'NONE',  ( -7.999999999999986677, 60.00000000000000711, 69.99999999999998579 ) ) ;
#6637=CARTESIAN_POINT ( 'NONE',  ( 0.8561741729129460632, 66.06698729999999387, 47.10000000109246798 ) ) ;
#6645=CARTESIAN_POINT ( 'NONE',  ( -2.500000000000001776, 64.00000000000000000, 49.99999999999999289 ) ) ;
#6655=CARTESIAN_POINT ( 'NONE',  ( -1.265664690411616068E-16, 66.06698730000000808, 45.55000000109246372 ) ) ;
#6663=VERTEX_POINT ( 'NONE', #7162 ) ;
#6671=CARTESIAN_POINT ( 'NONE',  ( -1.035533905932738863, 61.50000000000000000, 47.05000000218494449 ) ) ;
#6672=CARTESIAN_POINT ( 'NONE',  ( -7.999999999999986677, 68.00000000000000000, 45.00000000000000000 ) ) ;
#6682=CARTESIAN_POINT ( 'NONE',  ( 3.796994071234847710E-16, 61.93301269999999903, 48.95000000109246940 ) ) ;
#6693=PRODUCT_DEFINITION ( 'UNKNOWN', '', #17687, #16098 ) ;
#6719=CARTESIAN_POINT ( 'NONE',  ( 2.500000000000001776, 64.00000000000000000, 49.60000000000000142 ) ) ;
#6736=CARTESIAN_POINT ( 'NONE',  ( 0.8561741729129471734, 61.93301270000000613, 45.80000000109246372 ) ) ;
#6739=CARTESIAN_POINT ( 'NONE',  ( -1.035533905932738641, 66.50000000000000000, 49.85000000000000853 ) ) ;
#6741=CARTESIAN_POINT ( 'NONE',  ( -2.500000000000001776, 64.00000000000000000, 47.59999999999999432 ) ) ;
#6744=VERTEX_POINT ( 'NONE', #1387 ) ;
#6756=CARTESIAN_POINT ( 'NONE',  ( 1.035533905932739751, 61.50000000000000000, 48.75000000218494023 ) ) ;
#6769=EDGE_CURVE ( 'NONE', #3230, #9690, #12, .T. ) ;
#6771=CARTESIAN_POINT ( 'NONE',  ( -1.461580736456473906, 65.46158073645646880, 44.65000000109246514 ) ) ;
#6773=CARTESIAN_POINT ( 'NONE',  ( 3.796994071234847710E-16, 61.93301269999999903, 48.35000000109246798 ) ) ;
#6781=ORIENTED_EDGE ( 'NONE', *, *, #8780, .T. ) ;
#6792=CARTESIAN_POINT ( 'NONE',  ( -1.767766952966370209, 65.76776695296638309, 45.20000000218494307 ) ) ;
#6809=CARTESIAN_POINT ( 'NONE',  ( 1.035533905932738197, 66.50000000000000000, 46.65000000218494591 ) ) ;
#6814=CARTESIAN_POINT ( 'NONE',  ( -1.461580736456473462, 62.53841926354353120, 45.85000000109246798 ) ) ;
#6826=CARTESIAN_POINT ( 'NONE',  ( 1.461580736456473906, 62.53841926354353120, 45.85000000109246798 ) ) ;
#6829=CARTESIAN_POINT ( 'NONE',  ( -1.530808498934192803E-16, 66.50000000000000000, 49.79999999999999716 ) ) ;
#6837=ORIENTED_EDGE ( 'NONE', *, *, #3184, .F. ) ;
#6842=CARTESIAN_POINT ( 'NONE',  ( 1.035533905932738197, 66.50000000000000000, 48.25000000218493312 ) ) ;
#6850=CARTESIAN_POINT ( 'NONE',  ( -0.1365770217272186116, 61.93313928031658122, 44.99999999999987921 ) ) ;
#6854=CARTESIAN_POINT ( 'NONE',  ( 2.066987300000002303, 63.14382582708705627, 46.70000000109248361 ) ) ;
#6909=CARTESIAN_POINT ( 'NONE',  ( 4.592425496802577917E-16, 61.50000000000000000, 49.39999999999999147 ) ) ;
#6915=EDGE_CURVE ( 'NONE', #6744, #3230, #18351, .T. ) ;
#6916=CARTESIAN_POINT ( 'NONE',  ( 1.035533905932738197, 66.50000000000000000, 48.94999999999999574 ) ) ;
#6924=CARTESIAN_POINT ( 'NONE',  ( 1.461580736456473684, 65.46158073645646880, 46.85000000109246798 ) ) ;
#6927=CARTESIAN_POINT ( 'NONE',  ( 2.500000000000007550, 65.03553390593272354, 48.95000000218495018 ) ) ;
#6930=CARTESIAN_POINT ( 'NONE',  ( 2.500000000000001776, 64.00000000000000000, 47.99999999999999289 ) ) ;
#6942=CARTESIAN_POINT ( 'NONE',  ( 1.767766952966369987, 65.76776695296638309, 49.00000000218494023 ) ) ;
#6952=CARTESIAN_POINT ( 'NONE',  ( -1.461580736456473906, 65.46158073645646880, 46.25000000109247367 ) ) ;
#6954=CARTESIAN_POINT ( 'NONE',  ( 2.500000000000011102, 62.96446609406727646, 49.54999999999999716 ) ) ;
#6958=EDGE_CURVE ( 'NONE', #6663, #14186, #15000, .T. ) ;
#6972=ORIENTED_EDGE ( 'NONE', *, *, #8125, .T. ) ;
#6977=( BOUNDED_CURVE ( )  B_SPLINE_CURVE ( 2, ( #9097, #470, #18423, #12129, #7734, #3515, #1660, #2037, #16750 ),
 .UNSPECIFIED., .F., .F. ) 
 B_SPLINE_CURVE_WITH_KNOTS ( ( 3, 2, 2, 2, 3 ),
 ( 0.5714285714285711748, 0.5892857142857141906, 0.6071428571428569843, 0.6250000000000000000, 0.6428571428571429047 ),
 .UNSPECIFIED. ) 
 CURVE ( )  GEOMETRIC_REPRESENTATION_ITEM ( )  RATIONAL_B_SPLINE_CURVE ( ( 1.000000000000000888, 0.9238795325112857393, 1.000000000000000000, 0.9238795325112867385, 1.000000000000000000, 0.9238795325112867385, 1.000000000000000000, 0.9238795325112867385, 1.000000000000000000 ) ) 
 REPRESENTATION_ITEM ( '' )  );
#6982=CARTESIAN_POINT ( 'NONE',  ( -2.283493650000001818, 64.00000000000000000, 49.87500000054622973 ) ) ;
#7002=CARTESIAN_POINT ( 'NONE',  ( -0.8561741729129465073, 61.93301270000000613, 45.10000000109246798 ) ) ;
#7015=CARTESIAN_POINT ( 'NONE',  ( -2.066987300000000971, 63.14382582708704916, 46.40000000109247225 ) ) ;
#7018=CARTESIAN_POINT ( 'NONE',  ( 2.500000000000001776, 64.00000000000000000, 48.90000000218494591 ) ) ;
#7026=ORIENTED_EDGE ( 'NONE', *, *, #17643, .T. ) ;
#7034=CARTESIAN_POINT ( 'NONE',  ( 2.500000000000001776, 64.00000000000000000, 46.50000000218494733 ) ) ;
#7044=CARTESIAN_POINT ( 'NONE',  ( -1.461580736456473462, 62.53841926354353120, 44.85000000109246798 ) ) ;
#7051=ORIENTED_EDGE ( 'NONE', *, *, #189, .T. ) ;
#7085=CARTESIAN_POINT ( 'NONE',  ( -2.500000000000001776, 64.00000000000000000, 48.39999999999999858 ) ) ;
#7092=DIRECTION ( 'NONE',  ( 0.000000000000000000, -1.000000000000000000, 0.000000000000000000 ) ) ;
#7099=CARTESIAN_POINT ( 'NONE',  ( 2.500000000000001776, 65.03553390593273775, 48.85000000000000142 ) ) ;
#7116=CARTESIAN_POINT ( 'NONE',  ( -1.461580736456473906, 65.46158073645646880, 49.65000000109246514 ) ) ;
#7131=CARTESIAN_POINT ( 'NONE',  ( 1.035533905932738197, 66.50000000000000000, 45.05000000218494449 ) ) ;
#7141=CARTESIAN_POINT ( 'NONE',  ( 2.066987300000001415, 64.00000000000000000, 46.75000000109247367 ) ) ;
#7143=CARTESIAN_POINT ( 'NONE',  ( -1.035533905932738863, 61.50000000000000000, 49.35000000000000853 ) ) ;
#7162=CARTESIAN_POINT ( 'NONE',  ( -2.500000000000001776, 64.00000000000000000, 47.59999999999999432 ) ) ;
#7178=CARTESIAN_POINT ( 'NONE',  ( 0.000000000000000000, 64.00000000000000000, 49.99999999999999289 ) ) ;
#7193=CARTESIAN_POINT ( 'NONE',  ( -2.500000000000000888, 62.96446609406726935, 45.24999999999999289 ) ) ;
#7205=AXIS2_PLACEMENT_3D ( 'NONE', #1886, #16988, #7871 ) ;
#7216=CARTESIAN_POINT ( 'NONE',  ( -0.8561741729129461742, 66.06698730000000808, 48.00000000109246656 ) ) ;
#7232=CARTESIAN_POINT ( 'NONE',  ( 2.066987300000002303, 63.14382582708705627, 49.10000000109246088 ) ) ;
#7243=CARTESIAN_POINT ( 'NONE',  ( 2.066987300000001859, 64.85617417291294373, 48.60000000109246798 ) ) ;
#7245=ADVANCED_FACE ( 'NONE', ( #2973 ), #9051, .F. ) ;
#7247=VECTOR ( 'NONE', #8204, 1000.000000000000000 ) ;
#7273=DIRECTION ( 'NONE',  ( 0.000000000000000000, -1.000000000000000000, 0.000000000000000000 ) ) ;
#7286=ORIENTED_EDGE ( 'NONE', *, *, #17408, .F. ) ;
#7295=CARTESIAN_POINT ( 'NONE',  ( -1.767766952966369765, 62.23223304703363112, 46.89999999999999858 ) ) ;
#7315=EDGE_LOOP ( 'NONE', ( #4879, #9012, #11065, #12605 ) ) ;
#7320=CARTESIAN_POINT ( 'NONE',  ( -1.530808498934192803E-16, 66.50000000000000000, 47.39999999999999858 ) ) ;
#7327=CARTESIAN_POINT ( 'NONE',  ( -2.500000000000001776, 64.00000000000000000, 44.50000000218494733 ) ) ;
#7336=CARTESIAN_POINT ( 'NONE',  ( -2.066987300000001415, 64.00000000000000000, 47.35000000109246798 ) ) ;
#7347=ORIENTED_EDGE ( 'NONE', *, *, #3184, .T. ) ;
#7380=CARTESIAN_POINT ( 'NONE',  ( -1.767766952966370209, 65.76776695296638309, 45.89999999999999858 ) ) ;
#7394=CARTESIAN_POINT ( 'NONE',  ( 2.500000000000002220, 62.96446609406726935, 46.34999999999999432 ) ) ;
#7400=CARTESIAN_POINT ( 'NONE',  ( -1.942750718018138034, 65.20191092753520934, 45.00000000000002132 ) ) ;
#7415=DIRECTION ( 'NONE',  ( -1.000000000000000000, 1.110223024625155752E-14, 0.000000000000000000 ) ) ;
#7427=CARTESIAN_POINT ( 'NONE',  ( -1.035533905932738863, 61.50000000000000000, 44.65000000218494591 ) ) ;
#7431=VERTEX_POINT ( 'NONE', #14046 ) ;
#7435=CARTESIAN_POINT ( 'NONE',  ( 3.796994071234847710E-16, 61.93301269999999903, 48.35000000109246798 ) ) ;
#7437=FACE_OUTER_BOUND ( 'NONE', #390, .T. ) ;
#7487=CARTESIAN_POINT ( 'NONE',  ( -1.767766952966369765, 62.23223304703363112, 47.69999999999999574 ) ) ;
#7490=EDGE_LOOP ( 'NONE', ( #10763, #8230, #3208, #8162 ) ) ;
#7510=CARTESIAN_POINT ( 'NONE',  ( -2.066987300000001415, 64.00000000000000000, 45.75000000109247367 ) ) ;
#7526=CARTESIAN_POINT ( 'NONE',  ( -1.767766952966370209, 65.76776695296638309, 48.29999999999999716 ) ) ;
#7527=CARTESIAN_POINT ( 'NONE',  ( 2.500000000000001776, 65.03553390593273775, 45.75000000218494023 ) ) ;
#7529=ORIENTED_EDGE ( 'NONE', *, *, #2786, .T. ) ;
#7537=CARTESIAN_POINT ( 'NONE',  ( -1.461580736456473462, 62.53841926354353120, 46.65000000109247225 ) ) ;
#7554=CLOSED_SHELL ( 'NONE', ( #16065, #10995, #8448, #18271, #14203, #8310, #8010, #9034, #7245, #907, #13847, #4379, #9352, #3043, #10698, #3891, #13246, #13345, #5432, #9714, #7837, #10064, #8638, #10035, #7954, #3255 ) ) ;
#7592=EDGE_CURVE ( 'NONE', #14201, #4122, #17367, .T. ) ;
#7593=CARTESIAN_POINT ( 'NONE',  ( 4.592425496802577917E-16, 61.50000000000000000, 45.39999999999999858 ) ) ;
#7599=CARTESIAN_POINT ( 'NONE',  ( -0.7262361202807413596, 66.33061197500782669, 45.00000000000001421 ) ) ;
#7614=CARTESIAN_POINT ( 'NONE',  ( -0.8561741729129466183, 61.93301270000000613, 45.90000000109247225 ) ) ;
#7622=CARTESIAN_POINT ( 'NONE',  ( 1.035533905932738197, 66.50000000000000000, 47.34999999999998721 ) ) ;
#7630=CARTESIAN_POINT ( 'NONE',  ( -0.8561741729129465073, 61.93301270000000613, 46.50000000109247367 ) ) ;
#7638=CARTESIAN_POINT ( 'NONE',  ( 3.796994071234847710E-16, 61.93301269999999903, 46.75000000109246656 ) ) ;
#7646=DIRECTION ( 'NONE',  ( 1.000000000000000000, 0.000000000000000000, 0.000000000000000000 ) ) ;
#7656=FACE_OUTER_BOUND ( 'NONE', #7717, .T. ) ;
#7661=CARTESIAN_POINT ( 'NONE',  ( 2.500000000000001776, 64.00000000000000000, 47.19999999999999574 ) ) ;
#7662=LINE ( 'NONE', #3149, #8797 ) ;
#7693=UNCERTAINTY_MEASURE_WITH_UNIT (LENGTH_MEASURE( 1.000000000000000082E-05 ), #8983, 'distance_accuracy_value', 'NONE');
#7712=CARTESIAN_POINT ( 'NONE',  ( -2.066987300000001415, 63.14382582708705627, 46.60000000109246088 ) ) ;
#7717=EDGE_LOOP ( 'NONE', ( #7347, #7026, #14354, #3323 ) ) ;
#7731=CARTESIAN_POINT ( 'NONE',  ( 1.461580736456473684, 65.46158073645646880, 46.05000000109246372 ) ) ;
#7734=CARTESIAN_POINT ( 'NONE',  ( -1.530808498934192803E-16, 66.50000000000000000, 45.90000000218494591 ) ) ;
#7737=CARTESIAN_POINT ( 'NONE',  ( 0.8561741729129460632, 66.06698730000000808, 49.30000000109246372 ) ) ;
#7740=CARTESIAN_POINT ( 'NONE',  ( 3.796994071234847710E-16, 61.93301269999999903, 45.15000000109247225 ) ) ;
#7809=CARTESIAN_POINT ( 'NONE',  ( 1.461580736456473906, 62.53841926354353120, 48.45000000109246940 ) ) ;
#7816=EDGE_CURVE ( 'NONE', #535, #8383, #7662, .T. ) ;
#7827=CARTESIAN_POINT ( 'NONE',  ( -1.461580736456473906, 65.46158073645646880, 47.85000000109246798 ) ) ;
#7835=CARTESIAN_POINT ( 'NONE',  ( -2.500000000000001776, 64.00000000000000000, 46.79999999999999716 ) ) ;
#7837=ADVANCED_FACE ( 'NONE', ( #12158 ), #16387, .F. ) ;
#7843=CARTESIAN_POINT ( 'NONE',  ( -1.767766952966369765, 62.23223304703363112, 45.40000000218494591 ) ) ;
#7846=ORIENTED_EDGE ( 'NONE', *, *, #10910, .F. ) ;
#7858=( LENGTH_UNIT ( ) NAMED_UNIT ( * ) SI_UNIT ( .MILLI., .METRE. ) );
#7867=CARTESIAN_POINT ( 'NONE',  ( -2.066987300000001415, 64.00000000000000000, 48.75000000109246656 ) ) ;
#7871=DIRECTION ( 'NONE',  ( -1.000000000000000000, 0.000000000000000000, 0.000000000000000000 ) ) ;
#7873=DIRECTION ( 'NONE',  ( -1.000000000000000000, 0.000000000000000000, 0.000000000000000000 ) ) ;
#7885=VECTOR ( 'NONE', #9906, 1000.000000000000000 ) ;
#7906=CARTESIAN_POINT ( 'NONE',  ( -7.999999999999986677, 60.00000000000000711, 45.00000000000000000 ) ) ;
#7914=CARTESIAN_POINT ( 'NONE',  ( 0.000000000000000000, 64.00000000000000000, 49.99999999999999289 ) ) ;
#7916=CARTESIAN_POINT ( 'NONE',  ( 2.066987300000001859, 64.85617417291294373, 49.40000000109246514 ) ) ;
#7928=CARTESIAN_POINT ( 'NONE',  ( 1.461580736456473906, 62.53841926354353120, 45.05000000109246372 ) ) ;
#7938=CARTESIAN_POINT ( 'NONE',  ( -0.8561741729129461742, 66.06698729999999387, 44.80000000109246372 ) ) ;
#7952=ORIENTED_EDGE ( 'NONE', *, *, #8308, .T. ) ;
#7954=ADVANCED_FACE ( 'NONE', ( #18451 ), #4124, .F. ) ;
#7963=CARTESIAN_POINT ( 'NONE',  ( 1.461580736456473684, 65.46158073645646880, 48.45000000109247651 ) ) ;
#7976=EDGE_CURVE ( 'NONE', #15072, #9572, #568, .T. ) ;
#8003=CARTESIAN_POINT ( 'NONE',  ( -1.035533905932738863, 61.50000000000000000, 46.95000000000000284 ) ) ;
#8009=VECTOR ( 'NONE', #14237, 1000.000000000000000 ) ;
#8010=ADVANCED_FACE ( 'NONE', ( #12526 ), #5094, .F. ) ;
#8012=CARTESIAN_POINT ( 'NONE',  ( -2.066987300000001415, 64.00000000000000000, 48.95000000109246940 ) ) ;
#8026=CARTESIAN_POINT ( 'NONE',  ( 2.066987300000002303, 63.14382582708705627, 46.70000000109248361 ) ) ;
#8031=CARTESIAN_POINT ( 'NONE',  ( 3.796994071234847710E-16, 61.93301269999999903, 48.15000000109247225 ) ) ;
#8033=CARTESIAN_POINT ( 'NONE',  ( -2.066987300000001859, 64.85617417291294373, 44.90000000109247225 ) ) ;
#8063=CARTESIAN_POINT ( 'NONE',  ( -1.461580736456473906, 65.46158073645646880, 49.45000000109246940 ) ) ;
#8068=CARTESIAN_POINT ( 'NONE',  ( 1.993043451197827665, 65.46727981049029665, 44.99999999999998579 ) ) ;
#8081=DIRECTION ( 'NONE',  ( -0.000000000000000000, -0.000000000000000000, -1.000000000000000000 ) ) ;
#8084=CARTESIAN_POINT ( 'NONE',  ( 4.999999999999993783, 68.00000000000000000, 69.99999999999998579 ) ) ;
#8096=CARTESIAN_POINT ( 'NONE',  ( -7.999999999999986677, 68.00000000000000000, 45.00000000000000000 ) ) ;
#8105=CARTESIAN_POINT ( 'NONE',  ( 3.796994071234847710E-16, 61.93301269999999903, 46.75000000109246656 ) ) ;
#8107=CIRCLE ( 'NONE', #19047, 2.500000000000001776 ) ;
#8116=ORIENTED_EDGE ( 'NONE', *, *, #7816, .T. ) ;
#8125=EDGE_CURVE ( 'NONE', #535, #5700, #6128, .T. ) ;
#8138=( BOUNDED_CURVE ( )  B_SPLINE_CURVE ( 2, ( #5909, #14831, #17874, #4447, #17969, #16397, #8940, #6015, #1604 ),
 .UNSPECIFIED., .F., .T. ) 
 B_SPLINE_CURVE_WITH_KNOTS ( ( 3, 2, 2, 2, 3 ),
 ( 0.2142857142857140795, 0.2321428571428570675, 0.2500000000000000000, 0.2678571428571429602, 0.2857142857142859205 ),
 .UNSPECIFIED. ) 
 CURVE ( )  GEOMETRIC_REPRESENTATION_ITEM ( )  RATIONAL_B_SPLINE_CURVE ( ( 1.000000000000000888, 0.9238795325112859613, 1.000000000000000000, 0.9238795325112867385, 1.000000000000000000, 0.9238795325112867385, 1.000000000000000000, 0.9238795325112857393, 1.000000000000000888 ) ) 
 REPRESENTATION_ITEM ( '' )  );
#8140=CARTESIAN_POINT ( 'NONE',  ( -1.035533905932738641, 66.50000000000000000, 47.55000000218494449 ) ) ;
#8145=SURFACE_SIDE_STYLE ('',( #12349 ) ) ;
#8154=CARTESIAN_POINT ( 'NONE',  ( -2.066987300000001415, 64.85617417291294373, 48.10000000109246798 ) ) ;
#8162=ORIENTED_EDGE ( 'NONE', *, *, #15550, .F. ) ;
#8179=EDGE_CURVE ( 'NONE', #14706, #18337, #11483, .T. ) ;
#8204=DIRECTION ( 'NONE',  ( 1.000000000000000000, 0.000000000000000000, 0.000000000000000000 ) ) ;
#8206=CARTESIAN_POINT ( 'NONE',  ( -2.066987300000001859, 64.85617417291294373, 44.90000000109247225 ) ) ;
#8224=CARTESIAN_POINT ( 'NONE',  ( 1.461580736456473684, 65.46158073645646880, 45.25000000109247367 ) ) ;
#8226=CARTESIAN_POINT ( 'NONE',  ( -2.500000000000001776, 64.00000000000000000, 49.99999999999999289 ) ) ;
#8230=ORIENTED_EDGE ( 'NONE', *, *, #7592, .T. ) ;
#8239=CARTESIAN_POINT ( 'NONE',  ( 1.035533905932738197, 66.50000000000000000, 49.05000000218495160 ) ) ;
#8248=CARTESIAN_POINT ( 'NONE',  ( -2.500000000000001776, 64.00000000000000000, 45.19999999999999574 ) ) ;
#8250=CARTESIAN_POINT ( 'NONE',  ( -2.066987300000000971, 63.14382582708704916, 49.00000000109246656 ) ) ;
#8258=( BOUNDED_SURFACE ( )  B_SPLINE_SURFACE ( 1, 2, ( 
 ( #18814, #2251, #3905, #3624, #863, #8239, #6942, #12911, #3715, #11063, #9873, #6756, #15584, #15867, #8324, #14206, #772, #12724, #14113, #9594, #5387, #6842, #12815, #13002, #14295, #2427, #18813, #18720, #5198, #8411, #18631, #2152, #15961, #11344, #14386, #8140, #18907, #11436, #5284, #17430, #687, #4000, #9959, #17336, #11155, #6671, #962, #2525, #14484, #17153, #5473, #12634, #8508, #1055, #11243, #19003, #7034, #17062, #17246, #9688, #15681, #3816, #9782, #15775, #2341, #2818, #17822, #8601, #4298, #13394, #1355, #7527, #5668, #11527, #10454, #11725, #17927, #1255, #2721, #10152, #5865, #11632, #16152, #8892, #4499, #7131, #11935, #13099, #14978, #17721, #5964, #10255, #1454, #7427, #16448, #19390, #7327, #13294, #3015, #14583, #19098 ),
 ( #8991, #19296, #14787, #8694, #5762, #1552, #13502, #14678, #11825, #7232, #4399, #1154, #5569, #10360, #13202, #16354, #17621, #4198, #17521, #16245, #2918, #19195, #8799, #14882, #10061, #4101, #16055, #2615, #1656, #18024, #13794, #9378, #16845, #467, #7827, #13594, #6165, #10851, #12026, #4694, #270, #4597, #9479, #12422, #374, #15083, #6063, #15179, #3407, #16947, #6455, #2033, #9094, #9191, #1747, #83, #3114, #8026, #10945, #10555, #10651, #7630, #18224, #6361, #180, #1841, #3511, #15272, #15372, #15465, #7731, #12125, #1946, #18120, #16654, #16544, #13693, #18420, #12324, #3219, #6258, #12223, #13891, #4800, #10749, #16746, #3318, #9286, #18320, #4890, #7928, #4986, #3597, #2576, #16199, #15913, #14441, #2476, #12517, #8464, #1104 ) ),
 .UNSPECIFIED., .F., .F., .F. ) 
 B_SPLINE_SURFACE_WITH_KNOTS ( ( 2, 2 ),
 ( 3, 2, 2, 2, 2, 2, 2, 2, 2, 2, 2, 2, 2, 2, 2, 2, 2, 2, 2, 2, 2, 2, 2, 2, 2, 2, 2, 2, 2, 2, 2, 2, 2, 2, 2, 2, 2, 2, 2, 2, 2, 2, 2, 2, 2, 2, 2, 2, 2, 2, 3 ),
 ( 0.000000000000000000, 1.000000000000000000 ),
 ( 0.000000000000000000, 0.01785714285714285615, 0.03571428571428571230, 0.05357142857142856845, 0.07142857142857142461, 0.08928571428571428770, 0.1071428571428571369, 0.1250000000000000000, 0.1428571428571428492, 0.1607142857142857262, 0.1785714285714285754, 0.1964285714285714246, 0.2142857142857142738, 0.2321428571428571508, 0.2500000000000000000, 0.2678571428571428492, 0.2857142857142856984, 0.3035714285714285476, 0.3214285714285714524, 0.3392857142857143016, 0.3571428571428571508, 0.3750000000000000000, 0.3928571428571428492, 0.4107142857142856984, 0.4285714285714285476, 0.4464285714285714524, 0.4642857142857143016, 0.4821428571428571508, 0.5000000000000000000, 0.5178571428571429047, 0.5357142857142856984, 0.5535714285714286031, 0.5714285714285713969, 0.5892857142857143016, 0.6071428571428570953, 0.6250000000000000000, 0.6428571428571429047, 0.6607142857142856984, 0.6785714285714286031, 0.6964285714285713969, 0.7142857142857143016, 0.7321428571428570953, 0.7500000000000000000, 0.7678571428571429047, 0.7857142857142856984, 0.8035714285714286031, 0.8214285714285713969, 0.8392857142857143016, 0.8571428571428570953, 0.8750000000000000000, 0.8928571428571429047 ),
 .UNSPECIFIED. ) 
 GEOMETRIC_REPRESENTATION_ITEM ( )  RATIONAL_B_SPLINE_SURFACE ( (
 ( 1.000000000000000000, 0.9238795325112867385, 1.000000000000000000, 0.9238795325112867385, 1.000000000000000000, 0.9238795325112867385, 1.000000000000000000, 0.9238795325112867385, 1.000000000000000000, 0.9238795325112867385, 1.000000000000000000, 0.9238795325112867385, 1.000000000000000000, 0.9238795325112867385, 1.000000000000000000, 0.9238795325112867385, 1.000000000000000000, 0.9238795325112867385, 1.000000000000000000, 0.9238795325112867385, 1.000000000000000000, 0.9238795325112867385, 1.000000000000000000, 0.9238795325112867385, 1.000000000000000000, 0.9238795325112867385, 1.000000000000000000, 0.9238795325112867385, 1.000000000000000000, 0.9238795325112867385, 1.000000000000000000, 0.9238795325112867385, 1.000000000000000000, 0.9238795325112867385, 1.000000000000000000, 0.9238795325112867385, 1.000000000000000000, 0.9238795325112867385, 1.000000000000000000, 0.9238795325112867385, 1.000000000000000000, 0.9238795325112867385, 1.000000000000000000, 0.9238795325112867385, 1.000000000000000000, 0.9238795325112867385, 1.000000000000000000, 0.9238795325112867385, 1.000000000000000000, 0.9238795325112867385, 1.000000000000000000, 0.9238795325112867385, 1.000000000000000000, 0.9238795325112867385, 1.000000000000000000, 0.9238795325112867385, 1.000000000000000000, 0.9238795325112867385, 1.000000000000000000, 0.9238795325112867385, 1.000000000000000000, 0.9238795325112867385, 1.000000000000000000, 0.9238795325112867385, 1.000000000000000000, 0.9238795325112867385, 1.000000000000000000, 0.9238795325112867385, 1.000000000000000000, 0.9238795325112867385, 1.000000000000000000, 0.9238795325112867385, 1.000000000000000000, 0.9238795325112867385, 1.000000000000000000, 0.9238795325112867385, 1.000000000000000000, 0.9238795325112867385, 1.000000000000000000, 0.9238795325112867385, 1.000000000000000000, 0.9238795325112867385, 1.000000000000000000, 0.9238795325112867385, 1.000000000000000000, 0.9238795325112867385, 1.000000000000000000, 0.9238795325112867385, 1.000000000000000000, 0.9238795325112867385, 1.000000000000000000, 0.9238795325112867385, 1.000000000000000000, 0.9238795325112867385, 1.000000000000000000, 0.9238795325112867385, 1.000000000000000000, 0.9238795325112867385, 1.000000000000000000, 0.9238795325112867385, 1.000000000000000000),
 ( 1.000000000000000000, 0.9238795325112867385, 1.000000000000000000, 0.9238795325112867385, 1.000000000000000000, 0.9238795325112867385, 1.000000000000000000, 0.9238795325112867385, 1.000000000000000000, 0.9238795325112867385, 1.000000000000000000, 0.9238795325112867385, 1.000000000000000000, 0.9238795325112867385, 1.000000000000000000, 0.9238795325112867385, 1.000000000000000000, 0.9238795325112867385, 1.000000000000000000, 0.9238795325112867385, 1.000000000000000000, 0.9238795325112867385, 1.000000000000000000, 0.9238795325112867385, 1.000000000000000000, 0.9238795325112867385, 1.000000000000000000, 0.9238795325112867385, 1.000000000000000000, 0.9238795325112867385, 1.000000000000000000, 0.9238795325112867385, 1.000000000000000000, 0.9238795325112867385, 1.000000000000000000, 0.9238795325112867385, 1.000000000000000000, 0.9238795325112867385, 1.000000000000000000, 0.9238795325112867385, 1.000000000000000000, 0.9238795325112867385, 1.000000000000000000, 0.9238795325112867385, 1.000000000000000000, 0.9238795325112867385, 1.000000000000000000, 0.9238795325112867385, 1.000000000000000000, 0.9238795325112867385, 1.000000000000000000, 0.9238795325112867385, 1.000000000000000000, 0.9238795325112867385, 1.000000000000000000, 0.9238795325112867385, 1.000000000000000000, 0.9238795325112867385, 1.000000000000000000, 0.9238795325112867385, 1.000000000000000000, 0.9238795325112867385, 1.000000000000000000, 0.9238795325112867385, 1.000000000000000000, 0.9238795325112867385, 1.000000000000000000, 0.9238795325112867385, 1.000000000000000000, 0.9238795325112867385, 1.000000000000000000, 0.9238795325112867385, 1.000000000000000000, 0.9238795325112867385, 1.000000000000000000, 0.9238795325112867385, 1.000000000000000000, 0.9238795325112867385, 1.000000000000000000, 0.9238795325112867385, 1.000000000000000000, 0.9238795325112867385, 1.000000000000000000, 0.9238795325112867385, 1.000000000000000000, 0.9238795325112867385, 1.000000000000000000, 0.9238795325112867385, 1.000000000000000000, 0.9238795325112867385, 1.000000000000000000, 0.9238795325112867385, 1.000000000000000000, 0.9238795325112867385, 1.000000000000000000, 0.9238795325112867385, 1.000000000000000000, 0.9238795325112867385, 1.000000000000000000, 0.9238795325112867385, 1.000000000000000000) ) ) 
 REPRESENTATION_ITEM ( '' )  SURFACE ( )  );
#8267=CARTESIAN_POINT ( 'NONE',  ( 1.767766984964166399, 65.76776692096858312, 45.00000000000000000 ) ) ;
#8272=CARTESIAN_POINT ( 'NONE',  ( 8.000000000000014211, 60.00000000000000711, 66.99999999999997158 ) ) ;
#8289=CARTESIAN_POINT ( 'NONE',  ( -1.035533905932738863, 61.50000000000000000, 48.54999999999999716 ) ) ;
#8308=EDGE_CURVE ( 'NONE', #535, #17001, #17703, .T. ) ;
#8310=ADVANCED_FACE ( 'NONE', ( #4482 ), #4282, .F. ) ;
#8319=ORIENTED_EDGE ( 'NONE', *, *, #17872, .T. ) ;
#8324=CARTESIAN_POINT ( 'NONE',  ( -1.767766952966369765, 62.23223304703363112, 48.60000000218494165 ) ) ;
#8325=CARTESIAN_POINT ( 'NONE',  ( -7.999999999999986677, 60.00000000000000711, 45.00000000000000000 ) ) ;
#8334=CARTESIAN_POINT ( 'NONE',  ( -2.066987300000001859, 64.85617417291294373, 46.30000000109247082 ) ) ;
#8337=CARTESIAN_POINT ( 'NONE',  ( -2.066987300000001415, 64.00000000000000000, 49.75000000109246656 ) ) ;
#8340=CARTESIAN_POINT ( 'NONE',  ( 11.00000000000003020, 60.00000000000000711, 63.99999999999994316 ) ) ;
#8345=ORIENTED_EDGE ( 'NONE', *, *, #15528, .T. ) ;
#8381=CARTESIAN_POINT ( 'NONE',  ( 2.500000000000001776, 65.03553390593273775, 49.64999999999999147 ) ) ;
#8383=VERTEX_POINT ( 'NONE', #18103 ) ;
#8392=CARTESIAN_POINT ( 'NONE',  ( -0.8561741729129461742, 66.06698730000000808, 47.80000000109247082 ) ) ;
#8403=EDGE_CURVE ( 'NONE', #14706, #10838, #994, .T. ) ;
#8411=CARTESIAN_POINT ( 'NONE',  ( -1.035533905932738863, 61.50000000000000000, 47.85000000218494165 ) ) ;
#8423=CARTESIAN_POINT ( 'NONE',  ( -0.8561741729129465073, 61.93301270000000613, 45.70000000109248361 ) ) ;
#8427=CARTESIAN_POINT ( 'NONE',  ( 1.609560293423944355, 62.54174113348394570, 45.00000000000002132 ) ) ;
#8448=ADVANCED_FACE ( 'NONE', ( #18500 ), #18208, .F. ) ;
#8449=LINE ( 'NONE', #14618, #8009 ) ;
#8464=CARTESIAN_POINT ( 'NONE',  ( -0.8561741729129461742, 66.06698729999999387, 44.60000000109246088 ) ) ;
#8477=CARTESIAN_POINT ( 'NONE',  ( 3.796994071234847710E-16, 61.93301269999999903, 45.15000000109247225 ) ) ;
#8491=CARTESIAN_POINT ( 'NONE',  ( -0.8561741729129466183, 61.93301270000000613, 47.30000000109247082 ) ) ;
#8496=CARTESIAN_POINT ( 'NONE',  ( 1.767766952966370653, 62.23223304703363112, 47.89999999999999858 ) ) ;
#8508=CARTESIAN_POINT ( 'NONE',  ( -1.530808498934192803E-16, 66.50000000000000000, 46.70000000218494307 ) ) ;
#8520=CARTESIAN_POINT ( 'NONE',  ( 2.066987300000001859, 64.85617417291294373, 46.00000000109246656 ) ) ;
#8524=CARTESIAN_POINT ( 'NONE',  ( 0.7910017786515960436, 62.09035273295529578, 44.99999999999998579 ) ) ;
#8526=ORIENTED_EDGE ( 'NONE', *, *, #13942, .F. ) ;
#8549=EDGE_CURVE ( 'NONE', #10801, #6744, #15640, .T. ) ;
#8569=CARTESIAN_POINT ( 'NONE',  ( -2.500000000000001776, 65.03553390593273775, 49.14999999999999858 ) ) ;
#8583=CARTESIAN_POINT ( 'NONE',  ( 1.461580736456473906, 62.53841926354353120, 46.65000000109247225 ) ) ;
#8601=CARTESIAN_POINT ( 'NONE',  ( -1.035533905932738641, 66.50000000000000000, 45.95000000218494307 ) ) ;
#8611=CARTESIAN_POINT ( 'NONE',  ( 2.066987300000001859, 64.85617417291294373, 49.40000000109246514 ) ) ;
#8627=AXIS2_PLACEMENT_3D ( 'NONE', #5656, #11619, #7415 ) ;
#8638=ADVANCED_FACE ( 'NONE', ( #16088 ), #5507, .T. ) ;
#8644=VERTEX_POINT ( 'NONE', #14621 ) ;
#8664=CARTESIAN_POINT ( 'NONE',  ( 2.500000000000001776, 64.00000000000000000, 46.39999999999999858 ) ) ;
#8694=CARTESIAN_POINT ( 'NONE',  ( -0.8561741729129461742, 66.06698729999999387, 49.40000000109247225 ) ) ;
#8700=PLANE ( 'NONE',  #13520 ) ;
#8703=CARTESIAN_POINT ( 'NONE',  ( 1.461580736456473906, 62.53841926354353120, 49.25000000109246656 ) ) ;
#8712=CARTESIAN_POINT ( 'NONE',  ( -1.767766952966370209, 65.76776695296638309, 45.09999999999999432 ) ) ;
#8745=VECTOR ( 'NONE', #3817, 1000.000000000000000 ) ;
#8757=CARTESIAN_POINT ( 'NONE',  ( -1.767766952966370209, 65.76776695296638309, 46.69999999999999574 ) ) ;
#8758=CARTESIAN_POINT ( 'NONE',  ( 2.500000000000001776, 64.00000000000000000, 45.59999999999999432 ) ) ;
#8772=CARTESIAN_POINT ( 'NONE',  ( -2.500000000000001776, 64.00000000000000000, 49.30000000218494449 ) ) ;
#8777=CARTESIAN_POINT ( 'NONE',  ( 0.8561741729129460632, 66.06698730000000808, 46.30000000109247082 ) ) ;
#8779=VECTOR ( 'NONE', #17505, 1000.000000000000000 ) ;
#8780=EDGE_CURVE ( 'NONE', #1682, #14847, #15525, .T. ) ;
#8787=FILL_AREA_STYLE_COLOUR ( '', #13681 ) ;
#8789=CARTESIAN_POINT ( 'NONE',  ( -2.500000000000001776, 64.00000000000000000, 47.59999999999999432 ) ) ;
#8791=ORIENTED_EDGE ( 'NONE', *, *, #13703, .T. ) ;
#8792=PRODUCT_DEFINITION_SHAPE ( 'NONE', 'NONE',  #6693 ) ;
#8797=VECTOR ( 'NONE', #3250, 1000.000000000000000 ) ;
#8799=CARTESIAN_POINT ( 'NONE',  ( 1.461580736456473684, 65.46158073645646880, 48.45000000109247651 ) ) ;
#8801=ORIENTED_EDGE ( 'NONE', *, *, #2786, .F. ) ;
#8809=CARTESIAN_POINT ( 'NONE',  ( -0.8561741729129461742, 66.06698729999999387, 47.20000000109247651 ) ) ;
#8860=CARTESIAN_POINT ( 'NONE',  ( -2.500000000000001776, 65.03553390593273775, 46.74999999999999289 ) ) ;
#8876=CARTESIAN_POINT ( 'NONE',  ( 2.500000000000001776, 64.00000000000000000, 49.60000000000000142 ) ) ;
#8892=CARTESIAN_POINT ( 'NONE',  ( -1.035533905932738641, 66.50000000000000000, 45.15000000218493881 ) ) ;
#8894=ORIENTED_EDGE ( 'NONE', *, *, #15756, .T. ) ;
#8904=CARTESIAN_POINT ( 'NONE',  ( -1.461580736456473906, 65.46158073645646880, 48.85000000109246798 ) ) ;
#8929=AXIS2_PLACEMENT_3D ( 'NONE', #11761, #113, #14714 ) ;
#8931=CARTESIAN_POINT ( 'NONE',  ( 1.767766952966370653, 62.23223304703363112, 46.40000000218494591 ) ) ;
#8940=CARTESIAN_POINT ( 'NONE',  ( -1.767766952966369765, 62.23223304703363112, 47.80000000218494449 ) ) ;
#8942=CARTESIAN_POINT ( 'NONE',  ( 2.500000000000001776, 65.03553390593273775, 45.64999999999999858 ) ) ;
#8957=CARTESIAN_POINT ( 'NONE',  ( -1.035533905932738863, 61.50000000000000000, 46.14999999999999858 ) ) ;
#8963=CARTESIAN_POINT ( 'NONE',  ( -1.530808498934192803E-16, 66.50000000000000000, 45.00000000000000000 ) ) ;
#8974=DIRECTION ( 'NONE',  ( -0.000000000000000000, -0.000000000000000000, -1.000000000000000000 ) ) ;
#8975=CARTESIAN_POINT ( 'NONE',  ( 2.066987300000001859, 63.14382582708704916, 45.30000000109246372 ) ) ;
#8983=( LENGTH_UNIT ( ) NAMED_UNIT ( * ) SI_UNIT ( .MILLI., .METRE. ) );
#8988=CARTESIAN_POINT ( 'NONE',  ( -2.500000000000001776, 64.00000000000000000, 48.50000000218494023 ) ) ;
#8991=CARTESIAN_POINT ( 'NONE',  ( -2.066987300000001415, 64.00000000000000000, 49.55000000109247082 ) ) ;
#9002=CARTESIAN_POINT ( 'NONE',  ( -0.8561741729129465073, 61.93301270000000613, 47.50000000109246656 ) ) ;
#9012=ORIENTED_EDGE ( 'NONE', *, *, #1210, .T. ) ;
#9024=DIRECTION ( 'NONE',  ( 0.000000000000000000, 0.000000000000000000, 1.000000000000000000 ) ) ;
#9034=ADVANCED_FACE ( 'NONE', ( #10888 ), #18648, .F. ) ;
#9051=CYLINDRICAL_SURFACE ( 'NONE', #345, 2.500000000000001776 ) ;
#9055=CARTESIAN_POINT ( 'NONE',  ( 1.767766952966369987, 65.76776695296638309, 47.29999999999999716 ) ) ;
#9078=CARTESIAN_POINT ( 'NONE',  ( -1.461580736456473906, 65.46158073645646880, 46.45000000109246940 ) ) ;
#9079=CARTESIAN_POINT ( 'NONE',  ( -2.066987300000001415, 64.00000000000000000, 49.75000000109246656 ) ) ;
#9094=CARTESIAN_POINT ( 'NONE',  ( -1.265664690411616068E-16, 66.06698730000000808, 46.95000000109246940 ) ) ;
#9097=CARTESIAN_POINT ( 'NONE',  ( -2.500000000000001776, 64.00000000000000000, 46.10000000218494165 ) ) ;
#9100=VERTEX_POINT ( 'NONE', #3729 ) ;
#9102=CARTESIAN_POINT ( 'NONE',  ( 2.500000000000001776, 64.00000000000000000, 46.50000000218494733 ) ) ;
#9103=CARTESIAN_POINT ( 'NONE',  ( -2.066987300000001859, 64.85617417291294373, 48.90000000109247225 ) ) ;
#9110=CARTESIAN_POINT ( 'NONE',  ( -1.035533905932738641, 66.50000000000000000, 45.04999999999999005 ) ) ;
#9145=CARTESIAN_POINT ( 'NONE',  ( 2.500000000000001776, 64.00000000000000000, 45.59999999999999432 ) ) ;
#9158=LINE ( 'NONE', #15332, #3638 ) ;
#9188=CARTESIAN_POINT ( 'NONE',  ( -2.499999999999999556, 62.96446609406726225, 48.55000000218494449 ) ) ;
#9191=CARTESIAN_POINT ( 'NONE',  ( 0.8561741729129460632, 66.06698729999999387, 46.90000000109247225 ) ) ;
#9200=DIRECTION ( 'NONE',  ( -1.000000000000000000, 0.000000000000000000, 0.000000000000000000 ) ) ;
#9205=ORIENTED_EDGE ( 'NONE', *, *, #3519, .T. ) ;
#9242=ORIENTED_EDGE ( 'NONE', *, *, #10546, .F. ) ;
#9271=CARTESIAN_POINT ( 'NONE',  ( 2.500000000000001776, 64.00000000000000000, 48.10000000218494165 ) ) ;
#9272=CARTESIAN_POINT ( 'NONE',  ( -2.066987300000001415, 63.14382582708705627, 48.20000000109247651 ) ) ;
#9281=EDGE_LOOP ( 'NONE', ( #3162, #6183, #12726, #18845 ) ) ;
#9286=CARTESIAN_POINT ( 'NONE',  ( 2.066987300000001859, 64.85617417291294373, 45.20000000109248361 ) ) ;
#9296=CARTESIAN_POINT ( 'NONE',  ( -2.066987300000001415, 63.14382582708705627, 45.00000000109246656 ) ) ;
#9320=CARTESIAN_POINT ( 'NONE',  ( 0.8561741729129460632, 66.06698729999999387, 48.50000000109246656 ) ) ;
#9341=EDGE_LOOP ( 'NONE', ( #18268, #16435, #3476, #986 ) ) ;
#9352=ADVANCED_FACE ( 'NONE', ( #7437, #6074 ), #13404, .T. ) ;
#9363=CARTESIAN_POINT ( 'NONE',  ( 3.796994071234847710E-16, 61.93301269999999903, 47.55000000109247082 ) ) ;
#9378=CARTESIAN_POINT ( 'NONE',  ( -2.066987300000001415, 63.14382582708705627, 48.00000000109246656 ) ) ;
#9384=CARTESIAN_POINT ( 'NONE',  ( -2.066987300000001415, 64.00000000000000000, 47.95000000109246940 ) ) ;
#9386=CARTESIAN_POINT ( 'NONE',  ( 3.796994071234847710E-16, 61.93301269999999903, 45.95000000109246940 ) ) ;
#9408=EDGE_LOOP ( 'NONE', ( #8345, #19359, #8894, #9875 ) ) ;
#9418=CARTESIAN_POINT ( 'NONE',  ( -0.8561741729129461742, 66.06698729999999387, 49.40000000109247225 ) ) ;
#9435=CARTESIAN_POINT ( 'NONE',  ( -1.909647267044692676, 63.20899822134837365, 45.00000000000000000 ) ) ;
#9467=CARTESIAN_POINT ( 'NONE',  ( 1.461580736456473906, 62.53841926354353120, 47.65000000109247225 ) ) ;
#9479=CARTESIAN_POINT ( 'NONE',  ( 1.461580736456473906, 62.53841926354353120, 47.45000000109246940 ) ) ;
#9482=DIRECTION ( 'NONE',  ( -1.000000000000000000, 0.000000000000000000, 0.000000000000000000 ) ) ;
#9484=PLANE ( 'NONE',  #5924 ) ;
#9498=( BOUNDED_CURVE ( )  B_SPLINE_CURVE ( 2, ( #17403, #4176, #3977, #17222, #10127, #6916, #15931, #18887, #839 ),
 .UNSPECIFIED., .F., .T. ) 
 B_SPLINE_CURVE_WITH_KNOTS ( ( 3, 2, 2, 2, 3 ),
 ( 0.1428571428571429047, 0.1607142857142857262, 0.1785714285714285476, 0.1964285714285713413, 0.2142857142857141350 ),
 .UNSPECIFIED. ) 
 CURVE ( )  GEOMETRIC_REPRESENTATION_ITEM ( )  RATIONAL_B_SPLINE_CURVE ( ( 0.9999999999999997780, 0.9238795325112869605, 1.000000000000000000, 0.9238795325112867385, 1.000000000000000000, 0.9238795325112867385, 1.000000000000000000, 0.9238795325112872936, 0.9999999999999994449 ) ) 
 REPRESENTATION_ITEM ( '' )  );
#9519=EDGE_LOOP ( 'NONE', ( #2066, #14199, #5986, #3337 ) ) ;
#9522=ORIENTED_EDGE ( 'NONE', *, *, #11376, .F. ) ;
#9559=CARTESIAN_POINT ( 'NONE',  ( 1.461580736456473684, 65.46158073645646880, 47.85000000109246798 ) ) ;
#9572=VERTEX_POINT ( 'NONE', #3702 ) ;
#9575=CARTESIAN_POINT ( 'NONE',  ( 2.066987300000001859, 63.14382582708704916, 48.30000000109247082 ) ) ;
#9578=CARTESIAN_POINT ( 'NONE',  ( 8.000000000000000000, 68.00000000000000000, 66.99999999999997158 ) ) ;
#9594=CARTESIAN_POINT ( 'NONE',  ( -1.035533905932738641, 66.50000000000000000, 48.35000000218494165 ) ) ;
#9595=LINE ( 'NONE', #6672, #13448 ) ;
#9609=CARTESIAN_POINT ( 'NONE',  ( 2.066987300000001415, 64.00000000000000000, 47.55000000109247082 ) ) ;
#9610=CARTESIAN_POINT ( 'NONE',  ( -0.8561741729129466183, 61.93301270000000613, 47.50000000109246656 ) ) ;
#9653=CARTESIAN_POINT ( 'NONE',  ( -2.066987300000001859, 64.85617417291294373, 47.30000000109247082 ) ) ;
#9671=CARTESIAN_POINT ( 'NONE',  ( -1.461580736456473906, 65.46158073645646880, 45.45000000109246940 ) ) ;
#9688=CARTESIAN_POINT ( 'NONE',  ( 1.035533905932739751, 61.50000000000000000, 46.35000000218493454 ) ) ;
#9690=VERTEX_POINT ( 'NONE', #9578 ) ;
#9699=CARTESIAN_POINT ( 'NONE',  ( 1.767766984964166399, 65.76776692096858312, 45.00000000000000000 ) ) ;
#9701=CARTESIAN_POINT ( 'NONE',  ( -2.066987300000001415, 64.00000000000000000, 49.55000000109247082 ) ) ;
#9702=CARTESIAN_POINT ( 'NONE',  ( -0.8561741729129466183, 61.93301270000000613, 49.10000000109246088 ) ) ;
#9714=ADVANCED_FACE ( 'NONE', ( #2140 ), #14098, .T. ) ;
#9723=FACE_OUTER_BOUND ( 'NONE', #9894, .T. ) ;
#9752=CARTESIAN_POINT ( 'NONE',  ( 1.461580736456473684, 65.46158073645646880, 45.45000000109246940 ) ) ;
#9766=CARTESIAN_POINT ( 'NONE',  ( 0.7910017786515960436, 62.09035273295529578, 44.99999999999998579 ) ) ;
#9782=CARTESIAN_POINT ( 'NONE',  ( -1.767766952966369765, 62.23223304703363112, 46.20000000218494307 ) ) ;
#9789=CARTESIAN_POINT ( 'NONE',  ( -1.654487106972472477, 62.73153187564108180, 45.00000000000000000 ) ) ;
#9793=CARTESIAN_POINT ( 'NONE',  ( 3.796994071234847710E-16, 61.93301269999999903, 45.75000000109247367 ) ) ;
#9794=CARTESIAN_POINT ( 'NONE',  ( -1.265664690411616068E-16, 66.06698730000000808, 47.95000000109246940 ) ) ;
#9796=CARTESIAN_POINT ( 'NONE',  ( 2.500000000000001776, 64.00000000000000000, 49.60000000000000142 ) ) ;
#9811=CARTESIAN_POINT ( 'NONE',  ( -4.999999999999980460, 68.00000000000000000, 69.99999999999998579 ) ) ;
#9816=LINE ( 'NONE', #2287, #11144 ) ;
#9822=EDGE_CURVE ( 'NONE', #14706, #535, #18709, .T. ) ;
#9836=CARTESIAN_POINT ( 'NONE',  ( -0.8561741729129461742, 66.06698729999999387, 45.60000000109246088 ) ) ;
#9866=ORIENTED_EDGE ( 'NONE', *, *, #7976, .T. ) ;
#9873=CARTESIAN_POINT ( 'NONE',  ( 1.767766952966370653, 62.23223304703363112, 48.80000000218494449 ) ) ;
#9875=ORIENTED_EDGE ( 'NONE', *, *, #2645, .T. ) ;
#9884=CARTESIAN_POINT ( 'NONE',  ( -1.265664690411616068E-16, 66.06698730000000808, 46.95000000109246940 ) ) ;
#9894=EDGE_LOOP ( 'NONE', ( #5464, #4923, #7051, #9205 ) ) ;
#9906=DIRECTION ( 'NONE',  ( -0.000000000000000000, -0.000000000000000000, -1.000000000000000000 ) ) ;
#9922=CARTESIAN_POINT ( 'NONE',  ( -2.500000000000001776, 64.00000000000000000, 46.90000000218494591 ) ) ;
#9927=CARTESIAN_POINT ( 'NONE',  ( -2.500000000000000888, 62.96446609406726935, 49.24999999999999289 ) ) ;
#9941=CARTESIAN_POINT ( 'NONE',  ( 3.796994071234847710E-16, 61.93301269999999903, 46.55000000109247082 ) ) ;
#9944=CARTESIAN_POINT ( 'NONE',  ( -2.500000000000001776, 65.03553390593273775, 49.25000000218494023 ) ) ;
#9945=CARTESIAN_POINT ( 'NONE',  ( -2.500000000000001776, 64.00000000000000000, 49.65000000109247225 ) ) ;
#9952=ORIENTED_EDGE ( 'NONE', *, *, #1210, .F. ) ;
#9959=CARTESIAN_POINT ( 'NONE',  ( 1.767766952966370653, 62.23223304703363112, 47.20000000218494307 ) ) ;
#9973=CARTESIAN_POINT ( 'NONE',  ( 1.461580736456473906, 62.53841926354353120, 46.65000000109247225 ) ) ;
#9976=CARTESIAN_POINT ( 'NONE',  ( 2.314278491784644842, 64.59068907927618852, 45.00000000000002842 ) ) ;
#9981=EDGE_LOOP ( 'NONE', ( #7286, #271, #7846, #9242 ) ) ;
#10027=CARTESIAN_POINT ( 'NONE',  ( -2.066987300000001415, 64.00000000000000000, 45.75000000109247367 ) ) ;
#10035=ADVANCED_FACE ( 'NONE', ( #10342 ), #17503, .F. ) ;
#10045=CARTESIAN_POINT ( 'NONE',  ( 3.796994071234847710E-16, 61.93301269999999903, 45.75000000109247367 ) ) ;
#10053=FILL_AREA_STYLE ('',( #8787 ) ) ;
#10061=CARTESIAN_POINT ( 'NONE',  ( 2.066987300000001415, 64.00000000000000000, 48.35000000109246798 ) ) ;
#10064=ADVANCED_FACE ( 'NONE', ( #13757 ), #6615, .F. ) ;
#10069=CARTESIAN_POINT ( 'NONE',  ( -0.5386384701873604408, 61.99983965256841856, 45.00000000000003553 ) ) ;
#10072=CARTESIAN_POINT ( 'NONE',  ( -2.066987300000001859, 64.85617417291294373, 47.10000000109246798 ) ) ;
#10120=CARTESIAN_POINT ( 'NONE',  ( -1.035533905932738863, 61.50000000000000000, 45.34999999999999432 ) ) ;
#10127=CARTESIAN_POINT ( 'NONE',  ( -1.530808498934192803E-16, 66.50000000000000000, 48.99999999999999289 ) ) ;
#10138=CARTESIAN_POINT ( 'NONE',  ( -0.8561741729129461742, 66.06698730000000808, 48.80000000109247082 ) ) ;
#10152=CARTESIAN_POINT ( 'NONE',  ( -2.500000000000000888, 62.96446609406726935, 45.35000000218493454 ) ) ;
#10161=CARTESIAN_POINT ( 'NONE',  ( -2.066987300000001859, 64.85617417291294373, 49.70000000109248361 ) ) ;
#10208=CARTESIAN_POINT ( 'NONE',  ( -1.767766952966369765, 62.23223304703363112, 48.49999999999999289 ) ) ;
#10225=CARTESIAN_POINT ( 'NONE',  ( 1.035533905932738197, 66.50000000000000000, 48.14999999999999858 ) ) ;
#10228=B_SPLINE_CURVE_WITH_KNOTS ( 'NONE', 3,
 ( #19011, #3723, #11443, #6850, #5576, #10069, #14214, #12822, #17437, #14591, #3823, #9789, #15970, #2348 ),
 .UNSPECIFIED., .F., .F.,
 ( 4, 2, 2, 2, 2, 2, 4 ),
 ( 1.446806763283639067E-16, 0.0008152643689841970439, 0.001222896553476223412, 0.001630528737968249889, 0.002038160922460276366, 0.002445793106952302842, 0.003261057475936356663 ),
 .UNSPECIFIED. ) ;
#10230=( BOUNDED_CURVE ( )  B_SPLINE_CURVE ( 2, ( #19048, #5430, #5086, #5722, #14533, #4047, #10208, #11388, #7085 ),
 .UNSPECIFIED., .F., .F. ) 
 B_SPLINE_CURVE_WITH_KNOTS ( ( 3, 2, 2, 2, 3 ),
 ( 0.2142857142857141350, 0.2321428571428569565, 0.2499999999999997224, 0.2678571428571425161, 0.2857142857142853098 ),
 .UNSPECIFIED. ) 
 CURVE ( )  GEOMETRIC_REPRESENTATION_ITEM ( )  RATIONAL_B_SPLINE_CURVE ( ( 1.000000000000000666, 0.9238795325112861834, 1.000000000000000000, 0.9238795325112867385, 1.000000000000000000, 0.9238795325112867385, 1.000000000000000000, 0.9238795325112884038, 0.9999999999999983347 ) ) 
 REPRESENTATION_ITEM ( '' )  );
#10242=CARTESIAN_POINT ( 'NONE',  ( 0.000000000000000000, 64.00000000000000000, 49.99999999999999289 ) ) ;
#10243=CARTESIAN_POINT ( 'NONE',  ( 2.066987300000001859, 63.14382582708704916, 49.30000000109246372 ) ) ;
#10255=CARTESIAN_POINT ( 'NONE',  ( 1.035533905932739751, 61.50000000000000000, 44.75000000218494023 ) ) ;
#10262=DIRECTION ( 'NONE',  ( 0.000000000000000000, -0.000000000000000000, -1.000000000000000000 ) ) ;
#10265=CARTESIAN_POINT ( 'NONE',  ( -2.066987300000001859, 64.85617417291294373, 47.30000000109247082 ) ) ;
#10273=CARTESIAN_POINT ( 'NONE',  ( -2.500000000000006661, 65.03553390593272354, 45.14999999999999858 ) ) ;
#10278=CARTESIAN_POINT ( 'NONE',  ( -1.767766952966369765, 62.23223304703363112, 47.00000000218494733 ) ) ;
#10304=CARTESIAN_POINT ( 'NONE',  ( -2.500000000000001776, 64.00000000000000000, 46.00000000000000000 ) ) ;
#10319=CARTESIAN_POINT ( 'NONE',  ( 1.767766952966369987, 65.76776695296638309, 46.49999999999999289 ) ) ;
#10335=CARTESIAN_POINT ( 'NONE',  ( 2.500000000000001776, 64.00000000000000000, 48.79999999999999716 ) ) ;
#10342=FACE_OUTER_BOUND ( 'NONE', #6065, .T. ) ;
#10360=CARTESIAN_POINT ( 'NONE',  ( -0.8561741729129465073, 61.93301270000000613, 48.90000000109247225 ) ) ;
#10369=CARTESIAN_POINT ( 'NONE',  ( 1.461580736456473906, 62.53841926354353120, 48.45000000109246940 ) ) ;
#10375=ORIENTED_EDGE ( 'NONE', *, *, #6504, .T. ) ;
#10416=CARTESIAN_POINT ( 'NONE',  ( -1.035533905932738641, 66.50000000000000000, 45.84999999999998721 ) ) ;
#10437=CARTESIAN_POINT ( 'NONE',  ( 3.796994071234847710E-16, 61.93301269999999903, 45.95000000109246940 ) ) ;
#10446=CARTESIAN_POINT ( 'NONE',  ( 2.500000000000006661, 65.03553390593272354, 47.24999999999998579 ) ) ;
#10454=CARTESIAN_POINT ( 'NONE',  ( 1.767766952966370653, 62.23223304703363112, 45.60000000218494165 ) ) ;
#10463=CARTESIAN_POINT ( 'NONE',  ( 0.8561741729129472844, 61.93301270000000613, 46.80000000109246372 ) ) ;
#10476=VECTOR ( 'NONE', #15631, 1000.000000000000000 ) ;
#10480=CARTESIAN_POINT ( 'NONE',  ( -1.035533905932738863, 61.50000000000000000, 47.05000000218494449 ) ) ;
#10491=DIRECTION ( 'NONE',  ( -1.000000000000000000, 0.000000000000000000, 0.000000000000000000 ) ) ;
#10517=CARTESIAN_POINT ( 'NONE',  ( 2.500000000000001776, 65.03553390593273775, 45.64999999999999147 ) ) ;
#10519=( BOUNDED_CURVE ( )  B_SPLINE_CURVE ( 2, ( #4710, #15283, #4904, #16856, #18235, #1855, #7843, #15386, #13807 ),
 .UNSPECIFIED., .F., .F. ) 
 B_SPLINE_CURVE_WITH_KNOTS ( ( 3, 2, 2, 2, 3 ),
 ( 0.6428571428571429047, 0.6607142857142856984, 0.6785714285714286031, 0.6964285714285712858, 0.7142857142857141906 ),
 .UNSPECIFIED. ) 
 CURVE ( )  GEOMETRIC_REPRESENTATION_ITEM ( )  RATIONAL_B_SPLINE_CURVE ( ( 1.000000000000000000, 0.9238795325112867385, 1.000000000000000000, 0.9238795325112867385, 1.000000000000000000, 0.9238795325112867385, 1.000000000000000000, 0.9238795325112871826, 0.9999999999999995559 ) ) 
 REPRESENTATION_ITEM ( '' )  );
#10520=ORIENTED_EDGE ( 'NONE', *, *, #18596, .F. ) ;
#10538=CARTESIAN_POINT ( 'NONE',  ( 0.8561741729129471734, 61.93301270000000613, 45.20000000109248361 ) ) ;
#10546=EDGE_CURVE ( 'NONE', #14616, #3630, #10228, .T. ) ;
#10552=CARTESIAN_POINT ( 'NONE',  ( -1.035533905932738863, 61.50000000000000000, 48.65000000218493881 ) ) ;
#10555=CARTESIAN_POINT ( 'NONE',  ( 0.8561741729129472844, 61.93301270000000613, 46.60000000109246088 ) ) ;
#10558=CYLINDRICAL_SURFACE ( 'NONE', #12861, 2.500000000000001776 ) ;
#10564=CARTESIAN_POINT ( 'NONE',  ( 0.8561741729129460632, 66.06698729999999387, 47.10000000109246798 ) ) ;
#10565=CARTESIAN_POINT ( 'NONE',  ( 0.000000000000000000, 0.000000000000000000, 45.00000000000000000 ) ) ;
#10583=ORIENTED_EDGE ( 'NONE', *, *, #4279, .F. ) ;
#10628=CARTESIAN_POINT ( 'NONE',  ( 5.000000000000007994, 60.00000000000000711, 69.99999999999998579 ) ) ;
#10631=( BOUNDED_CURVE ( )  B_SPLINE_CURVE ( 2, ( #6930, #18800, #8496, #15763, #11333, #2328, #15574, #761, #6741 ),
 .UNSPECIFIED., .F., .F. ) 
 B_SPLINE_CURVE_WITH_KNOTS ( ( 3, 2, 2, 2, 3 ),
 ( 0.3571428571428572618, 0.3750000000000000555, 0.3928571428571429047, 0.4107142857142856984, 0.4285714285714284921 ),
 .UNSPECIFIED. ) 
 CURVE ( )  GEOMETRIC_REPRESENTATION_ITEM ( )  RATIONAL_B_SPLINE_CURVE ( ( 0.9999999999999995559, 0.9238795325112871826, 1.000000000000000000, 0.9238795325112867385, 1.000000000000000000, 0.9238795325112867385, 1.000000000000000000, 0.9238795325112869605, 0.9999999999999997780 ) ) 
 REPRESENTATION_ITEM ( '' )  );
#10634=CARTESIAN_POINT ( 'NONE',  ( -1.461580736456473906, 65.46158073645646880, 45.65000000109247225 ) ) ;
#10651=CARTESIAN_POINT ( 'NONE',  ( 3.796994071234847710E-16, 61.93301269999999903, 46.55000000109247082 ) ) ;
#10657=ORIENTED_EDGE ( 'NONE', *, *, #4892, .F. ) ;
#10658=CARTESIAN_POINT ( 'NONE',  ( 0.8561741729129471734, 61.93301270000000613, 49.00000000109246656 ) ) ;
#10661=CARTESIAN_POINT ( 'NONE',  ( -1.461580736456473462, 62.53841926354353120, 49.05000000109247082 ) ) ;
#10664=CARTESIAN_POINT ( 'NONE',  ( 1.035533905932738197, 66.50000000000000000, 47.45000000218494307 ) ) ;
#10698=ADVANCED_FACE ( 'NONE', ( #6237 ), #8700, .T. ) ;
#10736=CARTESIAN_POINT ( 'NONE',  ( -0.8561741729129461742, 66.06698730000000808, 45.60000000109246798 ) ) ;
#10737=CARTESIAN_POINT ( 'NONE',  ( 2.066987300000002303, 63.14382582708705627, 47.70000000109247651 ) ) ;
#10739=ORIENTED_EDGE ( 'NONE', *, *, #4698, .F. ) ;
#10749=CARTESIAN_POINT ( 'NONE',  ( -1.265664690411616068E-16, 66.06698730000000808, 45.35000000109246798 ) ) ;
#10755=CARTESIAN_POINT ( 'NONE',  ( 1.461580736456473684, 65.46158073645646880, 48.45000000109247651 ) ) ;
#10757=CARTESIAN_POINT ( 'NONE',  ( -2.066987300000001859, 64.85617417291294373, 45.70000000109248361 ) ) ;
#10763=ORIENTED_EDGE ( 'NONE', *, *, #17851, .F. ) ;
#10769=PLANE ( 'NONE',  #331 ) ;
#10774=CARTESIAN_POINT ( 'NONE',  ( -1.035533905932738863, 61.50000000000000000, 45.34999999999998721 ) ) ;
#10787=CARTESIAN_POINT ( 'NONE',  ( -2.500000000000001776, 64.00000000000000000, 46.90000000218494591 ) ) ;
#10789=CARTESIAN_POINT ( 'NONE',  ( 1.767766984964166399, 65.76776692096858312, 45.00000000000000000 ) ) ;
#10797=EDGE_CURVE ( 'NONE', #8383, #574, #9498, .T. ) ;
#10801=VERTEX_POINT ( 'NONE', #15840 ) ;
#10808=DIRECTION ( 'NONE',  ( -1.734723475976807094E-15, 1.000000000000000000, 0.000000000000000000 ) ) ;
#10835=CARTESIAN_POINT ( 'NONE',  ( 2.499999999999992895, 65.03553390593275196, 48.15000000218495302 ) ) ;
#10836=CARTESIAN_POINT ( 'NONE',  ( 0.8561741729129472844, 61.93301270000000613, 48.40000000109247225 ) ) ;
#10838=VERTEX_POINT ( 'NONE', #12888 ) ;
#10851=CARTESIAN_POINT ( 'NONE',  ( 0.8561741729129460632, 66.06698729999999387, 47.70000000109248361 ) ) ;
#10857=CARTESIAN_POINT ( 'NONE',  ( -1.461580736456473462, 62.53841926354353120, 48.85000000109246798 ) ) ;
#10860=CARTESIAN_POINT ( 'NONE',  ( 2.066987300000002303, 63.14382582708705627, 45.30000000109247082 ) ) ;
#10881=CARTESIAN_POINT ( 'NONE',  ( 8.000000000000014211, 60.00000000000000711, 45.00000000000000000 ) ) ;
#10885=CARTESIAN_POINT ( 'NONE',  ( -0.8561741729129465073, 61.93301270000000613, 48.10000000109246798 ) ) ;
#10888=FACE_OUTER_BOUND ( 'NONE', #13737, .T. ) ;
#10910=EDGE_CURVE ( 'NONE', #3630, #17515, #4636, .T. ) ;
#10929=CARTESIAN_POINT ( 'NONE',  ( 2.066987300000001859, 64.85617417291294373, 47.80000000109247082 ) ) ;
#10945=CARTESIAN_POINT ( 'NONE',  ( 1.461580736456473906, 62.53841926354353120, 46.65000000109247225 ) ) ;
#10950=CARTESIAN_POINT ( 'NONE',  ( -1.461580736456473906, 65.46158073645646880, 48.65000000109247225 ) ) ;
#10956=EDGE_CURVE ( 'NONE', #13224, #15564, #8138, .T. ) ;
#10959=ORIENTED_EDGE ( 'NONE', *, *, #16548, .T. ) ;
#10980=CARTESIAN_POINT ( 'NONE',  ( 1.461580736456473906, 62.53841926354353120, 48.25000000109246656 ) ) ;
#10981=( GEOMETRIC_REPRESENTATION_CONTEXT ( 3 ) GLOBAL_UNCERTAINTY_ASSIGNED_CONTEXT ( ( #13761 ) ) GLOBAL_UNIT_ASSIGNED_CONTEXT ( ( #7858, #17067, #2063 ) ) REPRESENTATION_CONTEXT ( 'NONE', 'WORKASPACE' ) );
#10990=( BOUNDED_CURVE ( )  B_SPLINE_CURVE ( 2, ( #10304, #13548, #7380, #13645, #2963, #13352, #229, #8942, #9145 ),
 .UNSPECIFIED., .F., .F. ) 
 B_SPLINE_CURVE_WITH_KNOTS ( ( 3, 2, 2, 2, 3 ),
 ( 0.7142857142857141906, 0.7321428571428569843, 0.7500000000000000000, 0.7678571428571429047, 0.7857142857142856984 ),
 .UNSPECIFIED. ) 
 CURVE ( )  GEOMETRIC_REPRESENTATION_ITEM ( )  RATIONAL_B_SPLINE_CURVE ( ( 1.000000000000000444, 0.9238795325112862944, 1.000000000000000000, 0.9238795325112867385, 1.000000000000000000, 0.9238795325112867385, 1.000000000000000000, 0.9238795325112867385, 1.000000000000000000 ) ) 
 REPRESENTATION_ITEM ( '' )  );
#10995=ADVANCED_FACE ( 'NONE', ( #11975 ), #18073, .F. ) ;
#10999=AXIS2_PLACEMENT_3D ( 'NONE', #7914, #1827, #548 ) ;
#11021=CARTESIAN_POINT ( 'NONE',  ( 1.767766952966370653, 62.23223304703363112, 47.09999999999999432 ) ) ;
#11027=CARTESIAN_POINT ( 'NONE',  ( -0.8561741729129461742, 66.06698729999999387, 47.20000000109247651 ) ) ;
#11050=CARTESIAN_POINT ( 'NONE',  ( 0.000000000000000000, 64.00000000000000000, 49.99999999999999289 ) ) ;
#11063=CARTESIAN_POINT ( 'NONE',  ( 2.500000000000002220, 62.96446609406726935, 48.85000000218494165 ) ) ;
#11065=ORIENTED_EDGE ( 'NONE', *, *, #2293, .F. ) ;
#11077=CARTESIAN_POINT ( 'NONE',  ( 1.461580736456473684, 65.46158073645646880, 47.65000000109247225 ) ) ;
#11079=CARTESIAN_POINT ( 'NONE',  ( 0.8561741729129471734, 61.93301270000000613, 47.60000000109246798 ) ) ;
#11101=CARTESIAN_POINT ( 'NONE',  ( 1.035533905932738197, 66.50000000000000000, 46.54999999999999716 ) ) ;
#11124=CARTESIAN_POINT ( 'NONE',  ( -0.8561741729129461742, 66.06698729999999387, 48.00000000109246656 ) ) ;
#11139=CARTESIAN_POINT ( 'NONE',  ( -1.461580736456473906, 65.46158073645646880, 46.25000000109247367 ) ) ;
#11141=CARTESIAN_POINT ( 'NONE',  ( 2.066987300000001415, 64.00000000000000000, 45.35000000109246798 ) ) ;
#11144=VECTOR ( 'NONE', #812, 1000.000000000000000 ) ;
#11155=CARTESIAN_POINT ( 'NONE',  ( 4.592425496802577917E-16, 61.50000000000000000, 47.10000000218494165 ) ) ;
#11167=CARTESIAN_POINT ( 'NONE',  ( 1.461580736456473684, 65.46158073645646880, 49.25000000109246656 ) ) ;
#11168=CARTESIAN_POINT ( 'NONE',  ( -0.8561741729129466183, 61.93301270000000613, 46.70000000109248361 ) ) ;
#11171=CARTESIAN_POINT ( 'NONE',  ( 2.224021093614878986, 63.47751682961200004, 45.00000000000000711 ) ) ;
#11173=VERTEX_POINT ( 'NONE', #17720 ) ;
#11209=CARTESIAN_POINT ( 'NONE',  ( 2.066987300000002303, 63.14382582708705627, 45.30000000109247082 ) ) ;
#11225=CARTESIAN_POINT ( 'NONE',  ( 1.170854245699165075, 62.24769277278622326, 45.02598915381526012 ) ) ;
#11227=CARTESIAN_POINT ( 'NONE',  ( -1.767766952966370209, 65.76776695296638309, 49.20000000218494307 ) ) ;
#11243=CARTESIAN_POINT ( 'NONE',  ( 1.767766952966369987, 65.76776695296638309, 46.60000000218494165 ) ) ;
#11256=CARTESIAN_POINT ( 'NONE',  ( -1.461580736456473462, 62.53841926354353120, 46.45000000109246940 ) ) ;
#11257=CARTESIAN_POINT ( 'NONE',  ( 2.066987300000001415, 64.00000000000000000, 49.35000000109246798 ) ) ;
#11313=EDGE_CURVE ( 'NONE', #8644, #2362, #16135, .T. ) ;
#11314=CARTESIAN_POINT ( 'NONE',  ( -1.530808498934192803E-16, 66.50000000000000000, 49.79999999999999716 ) ) ;
#11326=CARTESIAN_POINT ( 'NONE',  ( 2.500000000000001776, 64.00000000000000000, 49.99999999999999289 ) ) ;
#11328=CARTESIAN_POINT ( 'NONE',  ( -2.066987300000000971, 63.14382582708704916, 47.20000000109248361 ) ) ;
#11333=CARTESIAN_POINT ( 'NONE',  ( 4.592425496802577917E-16, 61.50000000000000000, 47.79999999999999716 ) ) ;
#11344=CARTESIAN_POINT ( 'NONE',  ( -2.500000000000001776, 65.03553390593273775, 47.65000000218494591 ) ) ;
#11354=CARTESIAN_POINT ( 'NONE',  ( 3.796994071234847710E-16, 61.93301269999999903, 44.95000000109246940 ) ) ;
#11376=EDGE_CURVE ( 'NONE', #15564, #6663, #6062, .T. ) ;
#11388=CARTESIAN_POINT ( 'NONE',  ( -2.499999999999984013, 62.96446609406724804, 48.45000000000000284 ) ) ;
#11399=CARTESIAN_POINT ( 'NONE',  ( -2.066987300000001859, 64.85617417291294373, 45.70000000109248361 ) ) ;
#11417=CARTESIAN_POINT ( 'NONE',  ( -1.265664690411616068E-16, 66.06698730000000808, 46.15000000109247225 ) ) ;
#11436=CARTESIAN_POINT ( 'NONE',  ( 1.035533905932738197, 66.50000000000000000, 47.45000000218495018 ) ) ;
#11443=CARTESIAN_POINT ( 'NONE',  ( 0.2673660800788628111, 61.93276224060318214, 44.99999999999988631 ) ) ;
#11447=CARTESIAN_POINT ( 'NONE',  ( 2.066987300000002303, 63.14382582708705627, 45.90000000109247225 ) ) ;
#11450=CARTESIAN_POINT ( 'NONE',  ( 1.035533905932739751, 61.50000000000000000, 49.44999999999999574 ) ) ;
#11483=( BOUNDED_CURVE ( )  B_SPLINE_CURVE ( 2, ( #8226, #13080, #14191, #6739, #6829, #11810, #13484, #19278, #8876 ),
 .UNSPECIFIED., .F., .F. ) 
 B_SPLINE_CURVE_WITH_KNOTS ( ( 3, 2, 2, 2, 3 ),
 ( 0.000000000000000000, 0.01785714285714280411, 0.03571428571428560822, 0.05357142857142841580, 0.07142857142857121644 ),
 .UNSPECIFIED. ) 
 CURVE ( )  GEOMETRIC_REPRESENTATION_ITEM ( )  RATIONAL_B_SPLINE_CURVE ( ( 1.000000000000000000, 0.9238795325112867385, 1.000000000000000000, 0.9238795325112867385, 1.000000000000000000, 0.9238795325112867385, 1.000000000000000000, 0.9238795325112876267, 0.9999999999999991118 ) ) 
 REPRESENTATION_ITEM ( '' )  );
#11490=DIRECTION ( 'NONE',  ( -1.000000000000000000, 0.000000000000000000, 0.000000000000000000 ) ) ;
#11496=CARTESIAN_POINT ( 'NONE',  ( 2.066987300000001415, 64.00000000000000000, 46.15000000109247225 ) ) ;
#11507=CARTESIAN_POINT ( 'NONE',  ( -2.066987300000001415, 64.00000000000000000, 47.15000000109247225 ) ) ;
#11527=CARTESIAN_POINT ( 'NONE',  ( 2.500000000000002220, 62.96446609406726935, 45.65000000218494591 ) ) ;
#11528=FACE_OUTER_BOUND ( 'NONE', #85, .T. ) ;
#11530=CARTESIAN_POINT ( 'NONE',  ( 2.500000000000001776, 64.00000000000000000, 45.59999999999999432 ) ) ;
#11538=CARTESIAN_POINT ( 'NONE',  ( -2.066987300000001415, 63.14382582708705627, 45.60000000109246088 ) ) ;
#11595=CARTESIAN_POINT ( 'NONE',  ( 1.461580736456473906, 62.53841926354353120, 45.25000000109247367 ) ) ;
#11616=CARTESIAN_POINT ( 'NONE',  ( -1.265664690411616068E-16, 66.06698730000000808, 47.15000000109247225 ) ) ;
#11619=DIRECTION ( 'NONE',  ( -0.000000000000000000, -0.000000000000000000, 1.000000000000000000 ) ) ;
#11632=CARTESIAN_POINT ( 'NONE',  ( -2.500000000000001776, 65.03553390593273775, 45.25000000218494733 ) ) ;
#11642=CARTESIAN_POINT ( 'NONE',  ( -1.461580736456473906, 65.46158073645646880, 49.65000000109246514 ) ) ;
#11693=CARTESIAN_POINT ( 'NONE',  ( -1.035533905932738863, 61.50000000000000000, 46.95000000000000995 ) ) ;
#11711=CARTESIAN_POINT ( 'NONE',  ( 0.8561741729129460632, 66.06698730000000808, 47.10000000109246798 ) ) ;
#11717=( NAMED_UNIT ( * ) PLANE_ANGLE_UNIT ( ) SI_UNIT ( $, .RADIAN. ) );
#11725=CARTESIAN_POINT ( 'NONE',  ( 1.035533905932739751, 61.50000000000000000, 45.55000000218493739 ) ) ;
#11728=CARTESIAN_POINT ( 'NONE',  ( 2.500000000000007105, 62.96446609406726225, 46.34999999999998721 ) ) ;
#11734=CARTESIAN_POINT ( 'NONE',  ( -1.461580736456473906, 65.46158073645646880, 46.45000000109246940 ) ) ;
#11761=CARTESIAN_POINT ( 'NONE',  ( 0.000000000000000000, 64.00000000000000000, 49.99999999999999289 ) ) ;
#11775=AXIS2_PLACEMENT_3D ( 'NONE', #15310, #15419, #7873 ) ;
#11795=CARTESIAN_POINT ( 'NONE',  ( 1.767766952966370653, 62.23223304703363112, 47.09999999999999432 ) ) ;
#11810=CARTESIAN_POINT ( 'NONE',  ( 1.035533905932738197, 66.50000000000000000, 49.74999999999998579 ) ) ;
#11825=CARTESIAN_POINT ( 'NONE',  ( 2.066987300000001415, 64.00000000000000000, 49.15000000109247225 ) ) ;
#11835=CARTESIAN_POINT ( 'NONE',  ( 1.461580736456473684, 65.46158073645646880, 48.65000000109247225 ) ) ;
#11895=CARTESIAN_POINT ( 'NONE',  ( 1.035533905932738197, 66.50000000000000000, 45.75000000000000000 ) ) ;
#11918=CARTESIAN_POINT ( 'NONE',  ( -0.8561741729129461742, 66.06698730000000808, 46.40000000109247225 ) ) ;
#11935=CARTESIAN_POINT ( 'NONE',  ( 1.767766952966369987, 65.76776695296638309, 45.00000000218494733 ) ) ;
#11944=CARTESIAN_POINT ( 'NONE',  ( 2.066987300000001859, 64.85617417291294373, 47.00000000109246656 ) ) ;
#11953=CARTESIAN_POINT ( 'NONE',  ( -2.500000000000001776, 64.00000000000000000, 45.19999999999999574 ) ) ;
#11975=FACE_OUTER_BOUND ( 'NONE', #9519, .T. ) ;
#11990=CARTESIAN_POINT ( 'NONE',  ( -1.035533905932738641, 66.50000000000000000, 48.24999999999999289 ) ) ;
#12007=CARTESIAN_POINT ( 'NONE',  ( -1.265664690411616068E-16, 66.06698730000000808, 45.55000000109246372 ) ) ;
#12017=SURFACE_SIDE_STYLE ('',( #16438 ) ) ;
#12018=ADVANCED_BREP_SHAPE_REPRESENTATION ( '', ( #3958, #1791 ), #12745 ) ;
#12025=CARTESIAN_POINT ( 'NONE',  ( 1.767766952966369987, 65.76776695296638309, 48.09999999999999432 ) ) ;
#12026=CARTESIAN_POINT ( 'NONE',  ( 1.461580736456473684, 65.46158073645646880, 47.65000000109247225 ) ) ;
#12027=ORIENTED_EDGE ( 'NONE', *, *, #19318, .T. ) ;
#12036=CARTESIAN_POINT ( 'NONE',  ( 0.8561741729129460632, 66.06698729999999387, 48.70000000109247651 ) ) ;
#12060=LINE ( 'NONE', #16184, #14880 ) ;
#12088=CARTESIAN_POINT ( 'NONE',  ( -1.530808498934192803E-16, 66.50000000000000000, 46.59999999999999432 ) ) ;
#12094=CARTESIAN_POINT ( 'NONE',  ( -1.366617256750952913, 65.93762474262220508, 45.00000000000000711 ) ) ;
#12108=CARTESIAN_POINT ( 'NONE',  ( 0.8561741729129460632, 66.06698729999999387, 49.50000000109246656 ) ) ;
#12125=CARTESIAN_POINT ( 'NONE',  ( 2.066987300000001859, 64.85617417291294373, 46.00000000109246656 ) ) ;
#12129=CARTESIAN_POINT ( 'NONE',  ( -1.035533905932738641, 66.50000000000000000, 45.95000000218494307 ) ) ;
#12136=CARTESIAN_POINT ( 'NONE',  ( 2.066987300000002303, 63.14382582708705627, 46.10000000109246798 ) ) ;
#12158=FACE_OUTER_BOUND ( 'NONE', #16075, .T. ) ;
#12185=VECTOR ( 'NONE', #6317, 1000.000000000000000 ) ;
#12186=CARTESIAN_POINT ( 'NONE',  ( -1.035533905932738641, 66.50000000000000000, 46.64999999999999858 ) ) ;
#12209=CARTESIAN_POINT ( 'NONE',  ( -2.066987300000001859, 64.85617417291294373, 46.50000000109246656 ) ) ;
#12223=CARTESIAN_POINT ( 'NONE',  ( -2.066987300000001859, 64.85617417291294373, 45.50000000109247367 ) ) ;
#12232=CARTESIAN_POINT ( 'NONE',  ( 1.461580736456473906, 62.53841926354353120, 48.25000000109246656 ) ) ;
#12266=CARTESIAN_POINT ( 'NONE',  ( 0.8561741729129460632, 66.06698729999999387, 49.30000000109246372 ) ) ;
#12292=CARTESIAN_POINT ( 'NONE',  ( 2.499999999999996447, 65.03553390593273775, 46.44999999999999574 ) ) ;
#12309=DIRECTION ( 'NONE',  ( 1.000000000000000000, 0.000000000000000000, 0.000000000000000000 ) ) ;
#12312=CARTESIAN_POINT ( 'NONE',  ( 1.461580736456473684, 65.46158073645646880, 46.25000000109246656 ) ) ;
#12324=CARTESIAN_POINT ( 'NONE',  ( -1.461580736456473462, 62.53841926354353120, 45.65000000109247225 ) ) ;
#12330=CARTESIAN_POINT ( 'NONE',  ( -0.8561741729129461742, 66.06698730000000808, 49.40000000109247225 ) ) ;
#12331=LINE ( 'NONE', #2138, #16259 ) ;
#12340=ORIENTED_EDGE ( 'NONE', *, *, #3536, .F. ) ;
#12349=SURFACE_STYLE_FILL_AREA ( #6580 ) ;
#12350=ORIENTED_EDGE ( 'NONE', *, *, #3297, .F. ) ;
#12358=CARTESIAN_POINT ( 'NONE',  ( -2.066987300000001859, 64.85617417291294373, 49.50000000109246656 ) ) ;
#12408=CARTESIAN_POINT ( 'NONE',  ( -0.8561741729129461742, 66.06698729999999387, 48.80000000109247082 ) ) ;
#12422=CARTESIAN_POINT ( 'NONE',  ( 0.8561741729129472844, 61.93301270000000613, 47.40000000109247225 ) ) ;
#12428=CARTESIAN_POINT ( 'NONE',  ( -0.8561741729129466183, 61.93301270000000613, 48.90000000109247225 ) ) ;
#12454=CARTESIAN_POINT ( 'NONE',  ( 0.8561741729129472844, 61.93301270000000613, 49.00000000109246656 ) ) ;
#12481=DIRECTION ( 'NONE',  ( -0.000000000000000000, -0.000000000000000000, -1.000000000000000000 ) ) ;
#12502=CARTESIAN_POINT ( 'NONE',  ( 3.796994071234847710E-16, 61.93301269999999903, 48.35000000109246798 ) ) ;
#12517=CARTESIAN_POINT ( 'NONE',  ( -1.461580736456473906, 65.46158073645646880, 44.65000000109246514 ) ) ;
#12524=CARTESIAN_POINT ( 'NONE',  ( 2.066987300000001415, 64.85617417291294373, 49.20000000109247651 ) ) ;
#12526=FACE_OUTER_BOUND ( 'NONE', #19087, .T. ) ;
#12547=SURFACE_STYLE_USAGE ( .BOTH. , #8145 ) ;
#12556=CARTESIAN_POINT ( 'NONE',  ( -2.066987300000001415, 64.00000000000000000, 47.95000000109246940 ) ) ;
#12558=COLOUR_RGB ( '', 0.31764706, 0.68627451, 0.89019608) ;
#12559=CARTESIAN_POINT ( 'NONE',  ( 0.8561741729129460632, 66.06698730000000808, 48.70000000109247651 ) ) ;
#12563=CARTESIAN_POINT ( 'NONE',  ( 2.161944888285726840, 65.13351296672139767, 44.99999999999997868 ) ) ;
#12602=CARTESIAN_POINT ( 'NONE',  ( 0.8561741729129472844, 61.93301270000000613, 49.20000000109247651 ) ) ;
#12605=ORIENTED_EDGE ( 'NONE', *, *, #6915, .T. ) ;
#12616=LINE ( 'NONE', #15276, #16327 ) ;
#12617=CARTESIAN_POINT ( 'NONE',  ( 1.461580736456473906, 62.53841926354353120, 47.45000000109246940 ) ) ;
#12634=CARTESIAN_POINT ( 'NONE',  ( -1.035533905932738641, 66.50000000000000000, 46.75000000218494733 ) ) ;
#12647=CARTESIAN_POINT ( 'NONE',  ( 1.461580736456473906, 62.53841926354353120, 47.45000000109246940 ) ) ;
#12648=CARTESIAN_POINT ( 'NONE',  ( -2.066987300000000971, 63.14382582708704916, 47.40000000109247225 ) ) ;
#12650=( BOUNDED_CURVE ( )  B_SPLINE_CURVE ( 2, ( #139, #2779, #8757, #12186, #17098, #11101, #531, #12292, #18477 ),
 .UNSPECIFIED., .F., .F. ) 
 B_SPLINE_CURVE_WITH_KNOTS ( ( 3, 2, 2, 2, 3 ),
 ( 0.5714285714285713969, 0.5892857142857143016, 0.6071428571428569843, 0.6249999999999998890, 0.6428571428571427937 ),
 .UNSPECIFIED. ) 
 CURVE ( )  GEOMETRIC_REPRESENTATION_ITEM ( )  RATIONAL_B_SPLINE_CURVE ( ( 1.000000000000000000, 0.9238795325112867385, 1.000000000000000000, 0.9238795325112867385, 1.000000000000000000, 0.9238795325112867385, 1.000000000000000000, 0.9238795325112871826, 0.9999999999999995559 ) ) 
 REPRESENTATION_ITEM ( '' )  );
#12652=CARTESIAN_POINT ( 'NONE',  ( 2.336476004967284137, 64.40336002165571472, 44.99999999999997868 ) ) ;
#12666=CARTESIAN_POINT ( 'NONE',  ( -2.500000000000006661, 65.03553390593272354, 45.25000000218494733 ) ) ;
#12672=DIRECTION ( 'NONE',  ( 1.000000000000000000, 0.000000000000000000, 0.000000000000000000 ) ) ;
#12675=LINE ( 'NONE', #1470, #13958 ) ;
#12691=CARTESIAN_POINT ( 'NONE',  ( 2.500000000000001776, 64.00000000000000000, 48.79999999999999716 ) ) ;
#12705=CARTESIAN_POINT ( 'NONE',  ( 0.8561741729129471734, 61.93301270000000613, 46.60000000109246798 ) ) ;
#12714=ORIENTED_EDGE ( 'NONE', *, *, #11313, .T. ) ;
#12724=CARTESIAN_POINT ( 'NONE',  ( -2.500000000000001776, 65.03553390593273775, 48.45000000218495018 ) ) ;
#12726=ORIENTED_EDGE ( 'NONE', *, *, #11376, .T. ) ;
#12727=EDGE_CURVE ( 'NONE', #4122, #5104, #16376, .T. ) ;
#12730=ORIENTED_EDGE ( 'NONE', *, *, #17408, .T. ) ;
#12737=CARTESIAN_POINT ( 'NONE',  ( -0.8561741729129461742, 66.06698729999999387, 45.40000000109246514 ) ) ;
#12738=CARTESIAN_POINT ( 'NONE',  ( -1.461580736456473462, 62.53841926354353120, 48.25000000109246656 ) ) ;
#12745=( GEOMETRIC_REPRESENTATION_CONTEXT ( 3 ) GLOBAL_UNCERTAINTY_ASSIGNED_CONTEXT ( ( #3762 ) ) GLOBAL_UNIT_ASSIGNED_CONTEXT ( ( #3707, #680, #14198 ) ) REPRESENTATION_CONTEXT ( 'NONE', 'WORKASPACE' ) );
#12778=DIRECTION ( 'NONE',  ( 1.000000000000000000, 0.000000000000000000, 0.000000000000000000 ) ) ;
#12780=CARTESIAN_POINT ( 'NONE',  ( -2.500000000000001776, 64.00000000000000000, 48.39999999999999858 ) ) ;
#12796=CARTESIAN_POINT ( 'NONE',  ( 2.066987300000001415, 64.00000000000000000, 46.75000000109247367 ) ) ;
#12800=CARTESIAN_POINT ( 'NONE',  ( -7.999999999999986677, 60.00000000000000711, 66.99999999999997158 ) ) ;
#12815=CARTESIAN_POINT ( 'NONE',  ( 1.767766952966369987, 65.76776695296638309, 48.20000000218494307 ) ) ;
#12822=CARTESIAN_POINT ( 'NONE',  ( -0.9169188819109246325, 62.14259808286531950, 45.00000000000001421 ) ) ;
#12827=CARTESIAN_POINT ( 'NONE',  ( 1.461580736456473684, 65.46158073645646880, 46.05000000109246372 ) ) ;
#12859=LINE ( 'NONE', #6982, #16808 ) ;
#12861=AXIS2_PLACEMENT_3D ( 'NONE', #6458, #6555, #9482 ) ;
#12881=CARTESIAN_POINT ( 'NONE',  ( -2.500000000000001776, 64.00000000000000000, 49.19999999999999574 ) ) ;
#12888=CARTESIAN_POINT ( 'NONE',  ( 2.500000000000001776, 64.00000000000000000, 49.99999999999999289 ) ) ;
#12895=CARTESIAN_POINT ( 'NONE',  ( -1.461580736456473906, 65.46158073645646880, 47.05000000109247082 ) ) ;
#12897=CARTESIAN_POINT ( 'NONE',  ( -1.035533905932738641, 66.50000000000000000, 49.15000000218494591 ) ) ;
#12911=CARTESIAN_POINT ( 'NONE',  ( 2.500000000000001776, 65.03553390593273775, 48.95000000218495018 ) ) ;
#12923=CARTESIAN_POINT ( 'NONE',  ( 0.8561741729129472844, 61.93301270000000613, 49.20000000109247651 ) ) ;
#12970=CARTESIAN_POINT ( 'NONE',  ( 1.767766952966369987, 65.76776695296638309, 48.89999999999999858 ) ) ;
#12974=( BOUNDED_CURVE ( )  B_SPLINE_CURVE ( 2, ( #6460, #382, #3605, #12330, #4993, #7737, #4702, #12524, #6264, #669, #4897, #10658, #473, #12428, #10857, #18126, #16852, #13699, #10950, #16660, #3413, #13996, #10755, #3225, #15471, #9575, #12232, #18231, #8031, #4806, #18524, #278, #9384, #566, #6557, #8392, #14367, #14564, #15848, #17411, #942, #15939, #12617, #5552, #17135, #8491, #12984, #11328, #11507, #2410, #12895, #17501, #845, #18984, #6924, #17231, #12796, #4078, #8583, #12705, #9941, #18894, #18706, #7015, #1136, #18612, #11139, #5456, #11417, #3983, #5178, #2506, #14468, #1040, #6826, #6736, #10045, #753, #16041, #2601, #15759, #3698, #9671, #15662, #2232, #18793, #8224, #14189, #3800, #5369, #5269, #11225, #9766 ),
 .UNSPECIFIED., .F., .F. ) 
 B_SPLINE_CURVE_WITH_KNOTS ( ( 3, 2, 2, 2, 2, 2, 2, 2, 2, 2, 2, 2, 2, 2, 2, 2, 2, 2, 2, 2, 2, 2, 2, 2, 2, 2, 2, 2, 2, 2, 2, 2, 2, 2, 2, 2, 2, 2, 2, 2, 2, 2, 2, 2, 2, 2, 3 ),
 ( 0.000000000000000000, 0.01785714285714285615, 0.03571428571428571230, 0.05357142857142856845, 0.07142857142857142461, 0.08928571428571428770, 0.1071428571428571369, 0.1250000000000000000, 0.1428571428571428492, 0.1607142857142857262, 0.1785714285714285754, 0.1964285714285714246, 0.2142857142857142738, 0.2321428571428571508, 0.2500000000000000000, 0.2678571428571428492, 0.2857142857142856984, 0.3035714285714285476, 0.3214285714285714524, 0.3392857142857143016, 0.3571428571428571508, 0.3750000000000000000, 0.3928571428571428492, 0.4107142857142856984, 0.4285714285714285476, 0.4464285714285714524, 0.4642857142857143016, 0.4821428571428571508, 0.5000000000000000000, 0.5178571428571429047, 0.5357142857142856984, 0.5535714285714286031, 0.5714285714285713969, 0.5892857142857143016, 0.6071428571428570953, 0.6250000000000000000, 0.6428571428571429047, 0.6607142857142856984, 0.6785714285714286031, 0.6964285714285713969, 0.7142857142857143016, 0.7321428571428570953, 0.7500000000000000000, 0.7678571428571429047, 0.7857142857142856984, 0.8035714285714286031, 0.8125000001876604427 ),
 .UNSPECIFIED. ) 
 CURVE ( )  GEOMETRIC_REPRESENTATION_ITEM ( )  RATIONAL_B_SPLINE_CURVE ( ( 1.000000000000000000, 0.9238795325112867385, 1.000000000000000000, 0.9238795325112867385, 1.000000000000000000, 0.9238795325112867385, 1.000000000000000000, 0.9238795325112867385, 1.000000000000000000, 0.9238795325112867385, 1.000000000000000000, 0.9238795325112867385, 1.000000000000000000, 0.9238795325112867385, 1.000000000000000000, 0.9238795325112867385, 1.000000000000000000, 0.9238795325112867385, 1.000000000000000000, 0.9238795325112867385, 1.000000000000000000, 0.9238795325112867385, 1.000000000000000000, 0.9238795325112867385, 1.000000000000000000, 0.9238795325112867385, 1.000000000000000000, 0.9238795325112867385, 1.000000000000000000, 0.9238795325112867385, 1.000000000000000000, 0.9238795325112867385, 1.000000000000000000, 0.9238795325112867385, 1.000000000000000000, 0.9238795325112867385, 1.000000000000000000, 0.9238795325112867385, 1.000000000000000000, 0.9238795325112867385, 1.000000000000000000, 0.9238795325112867385, 1.000000000000000000, 0.9238795325112867385, 1.000000000000000000, 0.9238795325112867385, 1.000000000000000000, 0.9238795325112867385, 1.000000000000000000, 0.9238795325112867385, 1.000000000000000000, 0.9238795325112867385, 1.000000000000000000, 0.9238795325112867385, 1.000000000000000000, 0.9238795325112867385, 1.000000000000000000, 0.9238795325112867385, 1.000000000000000000, 0.9238795325112867385, 1.000000000000000000, 0.9238795325112867385, 1.000000000000000000, 0.9238795325112867385, 1.000000000000000000, 0.9238795325112867385, 1.000000000000000000, 0.9238795325112867385, 1.000000000000000000, 0.9238795325112867385, 1.000000000000000000, 0.9238795325112867385, 1.000000000000000000, 0.9238795325112867385, 1.000000000000000000, 0.9238795325112867385, 1.000000000000000000, 0.9238795325112867385, 1.000000000000000000, 0.9238795325112867385, 1.000000000000000000, 0.9238795325112867385, 1.000000000000000000, 0.9238795325112867385, 1.000000000000000000, 0.9238795325112867385, 1.000000000000000000, 0.9238795325112867385, 1.000000000000000000, 0.9238795325112867385, 1.000000000000000000, 0.9619397654556944843, 0.9619397662556434803 ) ) 
 REPRESENTATION_ITEM ( '' )  );
#12984=CARTESIAN_POINT ( 'NONE',  ( -1.461580736456473462, 62.53841926354353120, 47.25000000109247367 ) ) ;
#12986=CARTESIAN_POINT ( 'NONE',  ( 1.035533905932738197, 66.50000000000000000, 49.05000000218495160 ) ) ;
#13002=CARTESIAN_POINT ( 'NONE',  ( 2.500000000000001776, 65.03553390593273775, 48.15000000218494591 ) ) ;
#13014=CARTESIAN_POINT ( 'NONE',  ( -1.265664690411616068E-16, 66.06698730000000808, 44.55000000109247082 ) ) ;
#13057=CARTESIAN_POINT ( 'NONE',  ( 0.000000000000000000, 64.00000000000000000, 49.99999999999999289 ) ) ;
#13064=CARTESIAN_POINT ( 'NONE',  ( 2.500000000000002220, 62.96446609406726935, 48.74999999999999289 ) ) ;
#13080=CARTESIAN_POINT ( 'NONE',  ( -2.500000000000001776, 65.03553390593273775, 49.94999999999998863 ) ) ;
#13081=CARTESIAN_POINT ( 'NONE',  ( 2.066987300000001415, 64.00000000000000000, 48.55000000109247082 ) ) ;
#13099=CARTESIAN_POINT ( 'NONE',  ( 2.500000000000001776, 65.03553390593273775, 44.95000000218494307 ) ) ;
#13109=CARTESIAN_POINT ( 'NONE',  ( 1.461580736456473906, 62.53841926354353120, 45.85000000109246798 ) ) ;
#13137=EDGE_CURVE ( 'NONE', #15072, #10801, #4572, .T. ) ;
#13158=CARTESIAN_POINT ( 'NONE',  ( 0.000000000000000000, 0.000000000000000000, 69.99999999999998579 ) ) ;
#13168=CARTESIAN_POINT ( 'NONE',  ( -1.767766952966370209, 65.76776695296638309, 48.29999999999999716 ) ) ;
#13187=CARTESIAN_POINT ( 'NONE',  ( -2.283493650000001818, 64.00000000000000000, 49.42500000163870766 ) ) ;
#13188=CARTESIAN_POINT ( 'NONE',  ( 0.8561741729129471734, 61.93301270000000613, 48.40000000109247225 ) ) ;
#13202=CARTESIAN_POINT ( 'NONE',  ( -1.461580736456473462, 62.53841926354353120, 48.85000000109246798 ) ) ;
#13214=CARTESIAN_POINT ( 'NONE',  ( 2.066987300000001859, 64.85617417291294373, 47.80000000109247082 ) ) ;
#13224=VERTEX_POINT ( 'NONE', #4866 ) ;
#13233=EDGE_LOOP ( 'NONE', ( #18955, #16214 ) ) ;
#13246=ADVANCED_FACE ( 'NONE', ( #637 ), #16921, .T. ) ;
#13249=DIRECTION ( 'NONE',  ( -0.000000000000000000, -0.000000000000000000, -1.000000000000000000 ) ) ;
#13261=CARTESIAN_POINT ( 'NONE',  ( -1.767766952966369765, 62.23223304703363112, 46.09999999999999432 ) ) ;
#13287=ORIENTED_EDGE ( 'NONE', *, *, #18855, .T. ) ;
#13294=CARTESIAN_POINT ( 'NONE',  ( -2.500000000000001776, 65.03553390593273775, 44.45000000218495018 ) ) ;
#13305=CARTESIAN_POINT ( 'NONE',  ( -2.066987300000001859, 64.85617417291294373, 48.10000000109246798 ) ) ;
#13321=CARTESIAN_POINT ( 'NONE',  ( 2.500000000000001776, 64.00000000000000000, 47.30000000218494449 ) ) ;
#13345=ADVANCED_FACE ( 'NONE', ( #17476 ), #5624, .F. ) ;
#13352=CARTESIAN_POINT ( 'NONE',  ( 1.035533905932738197, 66.50000000000000000, 45.75000000000000000 ) ) ;
#13365=CARTESIAN_POINT ( 'NONE',  ( -2.500000000000000888, 62.96446609406726935, 47.64999999999999858 ) ) ;
#13371=CARTESIAN_POINT ( 'NONE',  ( -0.3715438340500360481, 66.44684080192190834, 45.00000000000000711 ) ) ;
#13394=CARTESIAN_POINT ( 'NONE',  ( 1.035533905932738197, 66.50000000000000000, 45.85000000218494165 ) ) ;
#13403=CARTESIAN_POINT ( 'NONE',  ( 1.461580736456473906, 62.53841926354353120, 47.65000000109247225 ) ) ;
#13404=PLANE ( 'NONE',  #4407 ) ;
#13446=LINE ( 'NONE', #30, #14729 ) ;
#13448=VECTOR ( 'NONE', #491, 1000.000000000000000 ) ;
#13463=CARTESIAN_POINT ( 'NONE',  ( 1.767766952966369987, 65.76776695296638309, 48.09999999999999432 ) ) ;
#13471=CARTESIAN_POINT ( 'NONE',  ( -1.749252862646410556, 65.52426609366526122, 45.00000000000003553 ) ) ;
#13484=CARTESIAN_POINT ( 'NONE',  ( 1.767766952966369987, 65.76776695296638309, 49.69999999999999574 ) ) ;
#13486=CARTESIAN_POINT ( 'NONE',  ( 1.461580736456473906, 62.53841926354353120, 46.05000000109246372 ) ) ;
#13498=CARTESIAN_POINT ( 'NONE',  ( 2.499999999999996003, 62.96446609406726225, 48.85000000218494165 ) ) ;
#13502=CARTESIAN_POINT ( 'NONE',  ( 1.461580736456473684, 65.46158073645646880, 49.25000000109246656 ) ) ;
#13509=EDGE_LOOP ( 'NONE', ( #14144, #6373, #7952, #15522 ) ) ;
#13512=CARTESIAN_POINT ( 'NONE',  ( -0.8561741729129465073, 61.93301270000000613, 48.30000000109247082 ) ) ;
#13520=AXIS2_PLACEMENT_3D ( 'NONE', #3196, #4304, #10262 ) ;
#13536=CYLINDRICAL_SURFACE ( 'NONE', #8929, 2.500000000000001776 ) ;
#13548=CARTESIAN_POINT ( 'NONE',  ( -2.500000000000006661, 65.03553390593272354, 45.94999999999999574 ) ) ;
#13559=CARTESIAN_POINT ( 'NONE',  ( -2.500000000000001776, 65.03553390593273775, 47.54999999999999716 ) ) ;
#13578=CARTESIAN_POINT ( 'NONE',  ( 0.8561741729129460632, 66.06698730000000808, 45.50000000109247367 ) ) ;
#13594=CARTESIAN_POINT ( 'NONE',  ( -0.8561741729129461742, 66.06698729999999387, 47.80000000109247082 ) ) ;
#13605=CARTESIAN_POINT ( 'NONE',  ( 1.461580736456473684, 65.46158073645646880, 46.25000000109246656 ) ) ;
#13622=PLANE ( 'NONE',  #6310 ) ;
#13630=CARTESIAN_POINT ( 'NONE',  ( 0.000000000000000000, 64.00000000000000000, 49.99999999999999289 ) ) ;
#13645=CARTESIAN_POINT ( 'NONE',  ( -1.035533905932738641, 66.50000000000000000, 45.84999999999998721 ) ) ;
#13649=CARTESIAN_POINT ( 'NONE',  ( -18.99999999999997513, 68.00000000000000000, 55.99999999999995026 ) ) ;
#13678=CARTESIAN_POINT ( 'NONE',  ( -2.066987300000001415, 64.00000000000000000, 46.55000000109247082 ) ) ;
#13681=COLOUR_RGB ( '', 0.31764706, 0.68627451, 0.89019608) ;
#13693=CARTESIAN_POINT ( 'NONE',  ( 3.796994071234847710E-16, 61.93301269999999903, 45.75000000109247367 ) ) ;
#13699=CARTESIAN_POINT ( 'NONE',  ( -2.066987300000001415, 64.85617417291294373, 48.70000000109247651 ) ) ;
#13703=EDGE_CURVE ( 'NONE', #18046, #14186, #17095, .T. ) ;
#13704=APPLICATION_CONTEXT ( 'automotive_design' ) ;
#13713=CARTESIAN_POINT ( 'NONE',  ( 0.000000000000000000, 0.000000000000000000, 0.000000000000000000 ) ) ;
#13737=EDGE_LOOP ( 'NONE', ( #14304, #17954, #3408, #12714 ) ) ;
#13757=FACE_OUTER_BOUND ( 'NONE', #13233, .T. ) ;
#13761=UNCERTAINTY_MEASURE_WITH_UNIT (LENGTH_MEASURE( 1.000000000000000082E-05 ), #7858, 'distance_accuracy_value', 'NONE');
#13781=CARTESIAN_POINT ( 'NONE',  ( -1.461580736456473906, 65.46158073645646880, 47.25000000109246656 ) ) ;
#13794=CARTESIAN_POINT ( 'NONE',  ( -1.461580736456473462, 62.53841926354353120, 48.05000000109247082 ) ) ;
#13807=CARTESIAN_POINT ( 'NONE',  ( -2.500000000000001776, 64.00000000000000000, 45.30000000218493739 ) ) ;
#13812=CARTESIAN_POINT ( 'NONE',  ( 2.500000000000001776, 64.00000000000000000, 49.60000000000000142 ) ) ;
#13845=ORIENTED_EDGE ( 'NONE', *, *, #957, .T. ) ;
#13847=ADVANCED_FACE ( 'NONE', ( #9723 ), #15718, .F. ) ;
#13879=CARTESIAN_POINT ( 'NONE',  ( 2.066987300000002303, 63.14382582708705627, 48.50000000109246656 ) ) ;
#13891=CARTESIAN_POINT ( 'NONE',  ( -1.461580736456473906, 65.46158073645646880, 45.45000000109246940 ) ) ;
#13901=CARTESIAN_POINT ( 'NONE',  ( -1.035533905932738641, 66.50000000000000000, 47.55000000218494449 ) ) ;
#13923=DIRECTION ( 'NONE',  ( -1.734723475976807094E-15, 1.000000000000000000, 0.000000000000000000 ) ) ;
#13928=CARTESIAN_POINT ( 'NONE',  ( 3.796994071234847710E-16, 61.93301269999999903, 48.15000000109247225 ) ) ;
#13942=EDGE_CURVE ( 'NONE', #15953, #5501, #8449, .T. ) ;
#13946=B_SPLINE_CURVE_WITH_KNOTS ( 'NONE', 3,
 ( #10789, #6400, #8068, #12563, #5129, #9976, #12652, #5402, #14222, #11171, #3920, #2443, #14131, #8427, #18652, #980, #15979, #8524 ),
 .UNSPECIFIED., .F., .F.,
 ( 4, 2, 2, 2, 2, 2, 2, 2, 4 ),
 ( 0.000000000000000000, 0.0005599264810181958478, 0.001119852962036391696, 0.001679779443054587543, 0.002239705924072783391, 0.002799632405090979239, 0.003359558886109175087, 0.003919485367127341011, 0.004479411848145506067 ),
 .UNSPECIFIED. ) ;
#13951=DIRECTION ( 'NONE',  ( -0.000000000000000000, -0.000000000000000000, -1.000000000000000000 ) ) ;
#13958=VECTOR ( 'NONE', #19209, 1000.000000000000000 ) ;
#13968=CIRCLE ( 'NONE', #8627, 2.500000000000001776 ) ;
#13978=CARTESIAN_POINT ( 'NONE',  ( -2.066987300000001859, 64.85617417291294373, 48.90000000109247225 ) ) ;
#13979=CARTESIAN_POINT ( 'NONE',  ( -18.99999999999997513, 60.00000000000000711, 55.99999999999995026 ) ) ;
#13996=CARTESIAN_POINT ( 'NONE',  ( 0.8561741729129460632, 66.06698730000000808, 48.50000000109246656 ) ) ;
#13998=CARTESIAN_POINT ( 'NONE',  ( -1.265664690411616068E-16, 66.06698730000000808, 44.75000000109247367 ) ) ;
#14018=ORIENTED_EDGE ( 'NONE', *, *, #17489, .T. ) ;
#14023=CARTESIAN_POINT ( 'NONE',  ( -1.265664690411616068E-16, 66.06698730000000808, 47.75000000109246656 ) ) ;
#14025=CARTESIAN_POINT ( 'NONE',  ( 2.066987300000001415, 64.85617417291294373, 49.40000000109246514 ) ) ;
#14043=CARTESIAN_POINT ( 'NONE',  ( -2.500000000000001776, 64.00000000000000000, 48.50000000218494023 ) ) ;
#14044=CARTESIAN_POINT ( 'NONE',  ( 0.000000000000000000, 64.00000000000000000, 49.99999999999999289 ) ) ;
#14046=CARTESIAN_POINT ( 'NONE',  ( -2.500000000000001776, 64.00000000000000000, 46.00000000000000000 ) ) ;
#14074=CARTESIAN_POINT ( 'NONE',  ( -2.500000000000003109, 65.03553390593272354, 48.45000000218494307 ) ) ;
#14075=CARTESIAN_POINT ( 'NONE',  ( -2.066987300000001415, 63.14382582708705627, 49.00000000109246656 ) ) ;
#14097=VECTOR ( 'NONE', #7092, 1000.000000000000000 ) ;
#14098=PLANE ( 'NONE',  #16308 ) ;
#14113=CARTESIAN_POINT ( 'NONE',  ( -1.767766952966370209, 65.76776695296638309, 48.40000000218494591 ) ) ;
#14115=ORIENTED_EDGE ( 'NONE', *, *, #8549, .T. ) ;
#14125=CARTESIAN_POINT ( 'NONE',  ( -1.265664690411616068E-16, 66.06698730000000808, 49.35000000109246798 ) ) ;
#14127=CARTESIAN_POINT ( 'NONE',  ( 0.8561741729129460632, 66.06698730000000808, 47.90000000109247225 ) ) ;
#14131=CARTESIAN_POINT ( 'NONE',  ( 1.865360897248530714, 62.81633110618239613, 45.00000000000000711 ) ) ;
#14144=ORIENTED_EDGE ( 'NONE', *, *, #18596, .T. ) ;
#14169=CARTESIAN_POINT ( 'NONE',  ( 2.500000000000001776, 64.00000000000000000, 47.99999999999999289 ) ) ;
#14172=CARTESIAN_POINT ( 'NONE',  ( 1.035533905932739751, 61.50000000000000000, 48.64999999999999858 ) ) ;
#14177=EDGE_CURVE ( 'NONE', #1682, #663, #12060, .T. ) ;
#14186=VERTEX_POINT ( 'NONE', #7661 ) ;
#14189=CARTESIAN_POINT ( 'NONE',  ( 2.066987300000001415, 64.85617417291294373, 45.20000000109248361 ) ) ;
#14191=CARTESIAN_POINT ( 'NONE',  ( -1.767766952966370209, 65.76776695296638309, 49.89999999999999147 ) ) ;
#14198=( NAMED_UNIT ( * ) SI_UNIT ( $, .STERADIAN. ) SOLID_ANGLE_UNIT ( ) );
#14199=ORIENTED_EDGE ( 'NONE', *, *, #3536, .T. ) ;
#14201=VERTEX_POINT ( 'NONE', #15011 ) ;
#14203=ADVANCED_FACE ( 'NONE', ( #1588 ), #13536, .F. ) ;
#14206=CARTESIAN_POINT ( 'NONE',  ( -2.500000000000000888, 62.96446609406726935, 48.55000000218494449 ) ) ;
#14207=FACE_OUTER_BOUND ( 'NONE', #7315, .T. ) ;
#14214=CARTESIAN_POINT ( 'NONE',  ( -0.6673928701031922595, 62.03906428592985378, 45.00000000000002132 ) ) ;
#14217=CARTESIAN_POINT ( 'NONE',  ( 2.066987300000001859, 64.85617417291294373, 48.40000000109247225 ) ) ;
#14219=CARTESIAN_POINT ( 'NONE',  ( -2.066987300000001415, 64.85617417291294373, 48.90000000109247225 ) ) ;
#14221=CARTESIAN_POINT ( 'NONE',  ( 4.999999999999993783, 68.00000000000000000, 69.99999999999998579 ) ) ;
#14222=CARTESIAN_POINT ( 'NONE',  ( 2.314696032948281967, 63.84105539985402089, 44.99999999999999289 ) ) ;
#14237=DIRECTION ( 'NONE',  ( -0.000000000000000000, -0.000000000000000000, -1.000000000000000000 ) ) ;
#14239=AXIS2_PLACEMENT_3D ( 'NONE', #13158, #14538, #18767 ) ;
#14249=( BOUNDED_CURVE ( )  B_SPLINE_CURVE ( 2, ( #5968, #11728, #17930, #5672, #16248, #16550, #17627, #16451, #6067 ),
 .UNSPECIFIED., .F., .F. ) 
 B_SPLINE_CURVE_WITH_KNOTS ( ( 3, 2, 2, 2, 3 ),
 ( 0.6428571428571427937, 0.6607142857142855874, 0.6785714285714284921, 0.6964285714285712858, 0.7142857142857141906 ),
 .UNSPECIFIED. ) 
 CURVE ( )  GEOMETRIC_REPRESENTATION_ITEM ( )  RATIONAL_B_SPLINE_CURVE ( ( 1.000000000000000444, 0.9238795325112862944, 1.000000000000000000, 0.9238795325112867385, 1.000000000000000000, 0.9238795325112867385, 1.000000000000000000, 0.9238795325112871826, 0.9999999999999995559 ) ) 
 REPRESENTATION_ITEM ( '' )  );
#14261=CARTESIAN_POINT ( 'NONE',  ( -1.767766952966369765, 62.23223304703363112, 48.49999999999999289 ) ) ;
#14295=CARTESIAN_POINT ( 'NONE',  ( 2.500000000000001776, 64.00000000000000000, 48.10000000218494165 ) ) ;
#14304=ORIENTED_EDGE ( 'NONE', *, *, #18855, .F. ) ;
#14309=CARTESIAN_POINT ( 'NONE',  ( -0.8561741729129461742, 66.06698729999999387, 47.00000000109247367 ) ) ;
#14319=CARTESIAN_POINT ( 'NONE',  ( 2.500000000000001776, 64.00000000000000000, 48.90000000218494591 ) ) ;
#14346=CARTESIAN_POINT ( 'NONE',  ( -1.767766952966370209, 65.76776695296638309, 46.80000000218494449 ) ) ;
#14351=CARTESIAN_POINT ( 'NONE',  ( 1.461580736456473906, 62.53841926354353120, 46.05000000109246372 ) ) ;
#14354=ORIENTED_EDGE ( 'NONE', *, *, #7976, .F. ) ;
#14367=CARTESIAN_POINT ( 'NONE',  ( -1.265664690411616068E-16, 66.06698730000000808, 47.75000000109246656 ) ) ;
#14369=CARTESIAN_POINT ( 'NONE',  ( 1.767766952966369987, 65.76776695296638309, 49.00000000218494023 ) ) ;
#14380=EDGE_LOOP ( 'NONE', ( #1396, #3030, #12027, #1477 ) ) ;
#14386=CARTESIAN_POINT ( 'NONE',  ( -1.767766952966370209, 65.76776695296638309, 47.60000000218494165 ) ) ;
#14389=EDGE_CURVE ( 'NONE', #5700, #6405, #18044, .T. ) ;
#14399=CARTESIAN_POINT ( 'NONE',  ( 1.461580736456473684, 65.46158073645646880, 49.45000000109246940 ) ) ;
#14441=CARTESIAN_POINT ( 'NONE',  ( -2.066987300000001415, 64.00000000000000000, 44.75000000109247367 ) ) ;
#14454=CARTESIAN_POINT ( 'NONE',  ( -1.767766952966370209, 65.76776695296638309, 49.09999999999999432 ) ) ;
#14468=CARTESIAN_POINT ( 'NONE',  ( 2.066987300000001415, 64.00000000000000000, 45.95000000109246940 ) ) ;
#14480=ORIENTED_EDGE ( 'NONE', *, *, #8179, .T. ) ;
#14484=CARTESIAN_POINT ( 'NONE',  ( -2.500000000000001776, 64.00000000000000000, 46.90000000218494591 ) ) ;
#14494=CARTESIAN_POINT ( 'NONE',  ( -1.265664690411616068E-16, 66.06698730000000808, 45.35000000109246798 ) ) ;
#14522=CARTESIAN_POINT ( 'NONE',  ( -1.265664690411616068E-16, 66.06698730000000808, 47.15000000109247225 ) ) ;
#14533=CARTESIAN_POINT ( 'NONE',  ( 4.592425496802577917E-16, 61.50000000000000000, 48.59999999999999432 ) ) ;
#14538=DIRECTION ( 'NONE',  ( 0.000000000000000000, 0.000000000000000000, -1.000000000000000000 ) ) ;
#14539=LINE ( 'NONE', #14839, #14097 ) ;
#14548=CARTESIAN_POINT ( 'NONE',  ( -1.530808498934192803E-16, 66.50000000000000000, 48.99999999999999289 ) ) ;
#14563=VECTOR ( 'NONE', #1733, 1000.000000000000000 ) ;
#14564=CARTESIAN_POINT ( 'NONE',  ( 0.8561741729129460632, 66.06698730000000808, 47.70000000109248361 ) ) ;
#14567=CARTESIAN_POINT ( 'NONE',  ( -1.265664690411616068E-16, 66.06698730000000808, 49.55000000109247082 ) ) ;
#14576=VECTOR ( 'NONE', #15043, 1000.000000000000000 ) ;
#14583=CARTESIAN_POINT ( 'NONE',  ( -1.035533905932738641, 66.50000000000000000, 44.35000000218493454 ) ) ;
#14591=CARTESIAN_POINT ( 'NONE',  ( -1.262171526279624700, 62.35758450491420746, 45.00000000000000711 ) ) ;
#14595=CARTESIAN_POINT ( 'NONE',  ( -2.066987300000001415, 64.00000000000000000, 44.75000000109247367 ) ) ;
#14616=VERTEX_POINT ( 'NONE', #2030 ) ;
#14618=CARTESIAN_POINT ( 'NONE',  ( -2.500000000000001776, 64.00000000000000000, 49.99999999999999289 ) ) ;
#14621=CARTESIAN_POINT ( 'NONE',  ( -2.500000000000001776, 64.00000000000000000, 48.39999999999999858 ) ) ;
#14630=DIRECTION ( 'NONE',  ( -0.000000000000000000, -0.000000000000000000, -1.000000000000000000 ) ) ;
#14644=CARTESIAN_POINT ( 'NONE',  ( -2.500000000000001776, 64.00000000000000000, 47.59999999999999432 ) ) ;
#14662=CARTESIAN_POINT ( 'NONE',  ( 1.461580736456473906, 62.53841926354353120, 49.25000000109246656 ) ) ;
#14678=CARTESIAN_POINT ( 'NONE',  ( 2.066987300000001859, 64.85617417291294373, 49.20000000109247651 ) ) ;
#14688=CARTESIAN_POINT ( 'NONE',  ( -2.066987300000001415, 64.00000000000000000, 48.95000000109246940 ) ) ;
#14706=VERTEX_POINT ( 'NONE', #6645 ) ;
#14714=DIRECTION ( 'NONE',  ( -1.000000000000000000, 0.000000000000000000, 0.000000000000000000 ) ) ;
#14729=VECTOR ( 'NONE', #13249, 1000.000000000000000 ) ;
#14747=CARTESIAN_POINT ( 'NONE',  ( -2.500000000000001776, 64.00000000000000000, 45.19999999999999574 ) ) ;
#14770=CARTESIAN_POINT ( 'NONE',  ( -1.461580736456473462, 62.53841926354353120, 45.05000000109246372 ) ) ;
#14778=PRESENTATION_STYLE_ASSIGNMENT (( #19090 ) ) ;
#14787=CARTESIAN_POINT ( 'NONE',  ( -1.461580736456473906, 65.46158073645646880, 49.45000000109246940 ) ) ;
#14796=CARTESIAN_POINT ( 'NONE',  ( 0.8561741729129460632, 66.06698729999999387, 47.90000000109247225 ) ) ;
#14831=CARTESIAN_POINT ( 'NONE',  ( 2.500000000000010658, 62.96446609406726225, 48.05000000218495160 ) ) ;
#14839=CARTESIAN_POINT ( 'NONE',  ( -4.999999999999980460, 60.00000000000000711, 69.99999999999998579 ) ) ;
#14845=CARTESIAN_POINT ( 'NONE',  ( 2.500000000000001776, 65.03553390593273775, 46.45000000000000284 ) ) ;
#14847=VERTEX_POINT ( 'NONE', #5487 ) ;
#14860=EDGE_CURVE ( 'NONE', #18337, #8383, #16030, .T. ) ;
#14864=CARTESIAN_POINT ( 'NONE',  ( -2.066987300000000971, 63.14382582708704916, 46.60000000109246798 ) ) ;
#14880=VECTOR ( 'NONE', #16582, 1000.000000000000000 ) ;
#14882=CARTESIAN_POINT ( 'NONE',  ( 2.066987300000001859, 64.85617417291294373, 48.40000000109247225 ) ) ;
#14891=CARTESIAN_POINT ( 'NONE',  ( -1.461580736456473462, 62.53841926354353120, 48.25000000109246656 ) ) ;
#14946=CARTESIAN_POINT ( 'NONE',  ( 1.767766952966369987, 65.76776695296638309, 45.69999999999999574 ) ) ;
#14948=EDGE_CURVE ( 'NONE', #9100, #17922, #16832, .T. ) ;
#14958=CARTESIAN_POINT ( 'NONE',  ( 2.500000000000001776, 64.00000000000000000, 46.39999999999999858 ) ) ;
#14970=( NAMED_UNIT ( * ) SI_UNIT ( $, .STERADIAN. ) SOLID_ANGLE_UNIT ( ) );
#14978=CARTESIAN_POINT ( 'NONE',  ( 2.500000000000001776, 64.00000000000000000, 44.90000000218493881 ) ) ;
#14986=CARTESIAN_POINT ( 'NONE',  ( -1.265664690411616068E-16, 66.06698730000000808, 47.95000000109246940 ) ) ;
#15000=( BOUNDED_CURVE ( )  B_SPLINE_CURVE ( 2, ( #8789, #4192, #6056, #17615, #7320, #7622, #4391, #10446, #5858 ),
 .UNSPECIFIED., .F., .F. ) 
 B_SPLINE_CURVE_WITH_KNOTS ( ( 3, 2, 2, 2, 3 ),
 ( 0.4285714285714284921, 0.4464285714285714524, 0.4642857142857143016, 0.4821428571428572063, 0.5000000000000001110 ),
 .UNSPECIFIED. ) 
 CURVE ( )  GEOMETRIC_REPRESENTATION_ITEM ( )  RATIONAL_B_SPLINE_CURVE ( ( 1.000000000000000222, 0.9238795325112865164, 1.000000000000000000, 0.9238795325112867385, 1.000000000000000000, 0.9238795325112867385, 1.000000000000000000, 0.9238795325112862944, 1.000000000000000444 ) ) 
 REPRESENTATION_ITEM ( '' )  );
#15011=CARTESIAN_POINT ( 'NONE',  ( 2.500000000000001776, 64.00000000000000000, 45.70000000218494307 ) ) ;
#15042=CARTESIAN_POINT ( 'NONE',  ( -2.500000000000001776, 65.03553390593273775, 45.95000000000000995 ) ) ;
#15043=DIRECTION ( 'NONE',  ( -0.000000000000000000, -0.000000000000000000, -1.000000000000000000 ) ) ;
#15051=CARTESIAN_POINT ( 'NONE',  ( -2.019187605927083240, 65.02780627284310810, 45.00000000000004263 ) ) ;
#15066=CARTESIAN_POINT ( 'NONE',  ( -2.066987300000001859, 64.85617417291294373, 49.70000000109248361 ) ) ;
#15069=DIRECTION ( 'NONE',  ( -1.000000000000000000, 0.000000000000000000, 0.000000000000000000 ) ) ;
#15072=VERTEX_POINT ( 'NONE', #18694 ) ;
#15082=CARTESIAN_POINT ( 'NONE',  ( -1.530808498934192803E-16, 66.50000000000000000, 48.19999999999999574 ) ) ;
#15083=CARTESIAN_POINT ( 'NONE',  ( -0.8561741729129465073, 61.93301270000000613, 47.30000000109247082 ) ) ;
#15092=CARTESIAN_POINT ( 'NONE',  ( 2.066987300000001415, 64.00000000000000000, 48.55000000109247082 ) ) ;
#15093=APPLICATION_CONTEXT ( 'automotive_design' ) ;
#15133=ORIENTED_EDGE ( 'NONE', *, *, #189, .F. ) ;
#15137=DIRECTION ( 'NONE',  ( -0.000000000000000000, -0.000000000000000000, -1.000000000000000000 ) ) ;
#15142=DIRECTION ( 'NONE',  ( -1.000000000000000000, -0.000000000000000000, -0.000000000000000000 ) ) ;
#15179=CARTESIAN_POINT ( 'NONE',  ( -2.066987300000001415, 63.14382582708705627, 47.20000000109248361 ) ) ;
#15186=CARTESIAN_POINT ( 'NONE',  ( -4.999999999999980460, 0.000000000000000000, 69.99999999999998579 ) ) ;
#15223=DIRECTION ( 'NONE',  ( -0.000000000000000000, -0.000000000000000000, -1.000000000000000000 ) ) ;
#15258=CARTESIAN_POINT ( 'NONE',  ( -1.461580736456473462, 62.53841926354353120, 46.65000000109247225 ) ) ;
#15272=CARTESIAN_POINT ( 'NONE',  ( -0.8561741729129461742, 66.06698729999999387, 46.20000000109247651 ) ) ;
#15276=CARTESIAN_POINT ( 'NONE',  ( -2.500000000000001776, 64.00000000000000000, 49.99999999999999289 ) ) ;
#15281=CARTESIAN_POINT ( 'NONE',  ( 5.000000000000111910, 8.673617379884229532E-15, 69.99999999999998579 ) ) ;
#15283=CARTESIAN_POINT ( 'NONE',  ( 2.500000000000002220, 62.96446609406726225, 45.65000000218494591 ) ) ;
#15288=SHAPE_REPRESENTATION ( 'Lever Press Handle Knob', ( #1791 ), #12745 ) ;
#15310=CARTESIAN_POINT ( 'NONE',  ( 0.000000000000000000, 64.00000000000000000, 49.99999999999999289 ) ) ;
#15320=VECTOR ( 'NONE', #18449, 1000.000000000000000 ) ;
#15332=CARTESIAN_POINT ( 'NONE',  ( -7.999999999999986677, 68.00000000000000000, 69.99999999999998579 ) ) ;
#15347=CARTESIAN_POINT ( 'NONE',  ( 4.592425496802577917E-16, 61.50000000000000000, 46.99999999999999289 ) ) ;
#15354=CARTESIAN_POINT ( 'NONE',  ( 2.066987300000001415, 64.00000000000000000, 49.35000000109246798 ) ) ;
#15366=ORIENTED_EDGE ( 'NONE', *, *, #10910, .T. ) ;
#15372=CARTESIAN_POINT ( 'NONE',  ( -1.265664690411616068E-16, 66.06698730000000808, 46.15000000109247225 ) ) ;
#15383=CARTESIAN_POINT ( 'NONE',  ( -0.8561741729129461742, 66.06698729999999387, 45.60000000109246088 ) ) ;
#15386=CARTESIAN_POINT ( 'NONE',  ( -2.499999999999996003, 62.96446609406726225, 45.35000000218493454 ) ) ;
#15412=CARTESIAN_POINT ( 'NONE',  ( -2.066987300000001415, 63.14382582708705627, 48.80000000109247082 ) ) ;
#15419=DIRECTION ( 'NONE',  ( -0.000000000000000000, -0.000000000000000000, -1.000000000000000000 ) ) ;
#15453=CARTESIAN_POINT ( 'NONE',  ( -1.461580736456473462, 62.53841926354353120, 49.05000000109247082 ) ) ;
#15465=CARTESIAN_POINT ( 'NONE',  ( 0.8561741729129460632, 66.06698729999999387, 46.10000000109246798 ) ) ;
#15471=CARTESIAN_POINT ( 'NONE',  ( 2.066987300000001415, 64.00000000000000000, 48.35000000109246798 ) ) ;
#15484=ORIENTED_EDGE ( 'NONE', *, *, #8780, .F. ) ;
#15522=ORIENTED_EDGE ( 'NONE', *, *, #6386, .T. ) ;
#15525=( BOUNDED_CURVE ( )  B_SPLINE_CURVE ( 2, ( #316, #16489, #8931, #16786, #16390, #2953, #4638, #1494, #1687 ),
 .UNSPECIFIED., .F., .F. ) 
 B_SPLINE_CURVE_WITH_KNOTS ( ( 3, 2, 2, 2, 3 ),
 ( 0.4999999999999999445, 0.5178571428571427937, 0.5357142857142855874, 0.5535714285714283811, 0.5714285714285711748 ),
 .UNSPECIFIED. ) 
 CURVE ( )  GEOMETRIC_REPRESENTATION_ITEM ( )  RATIONAL_B_SPLINE_CURVE ( ( 1.000000000000000222, 0.9238795325112865164, 1.000000000000000000, 0.9238795325112867385, 1.000000000000000000, 0.9238795325112867385, 1.000000000000000000, 0.9238795325112877377, 0.9999999999999990008 ) ) 
 REPRESENTATION_ITEM ( '' )  );
#15528=EDGE_CURVE ( 'NONE', #16168, #6563, #9158, .T. ) ;
#15544=CARTESIAN_POINT ( 'NONE',  ( 1.035533905932739751, 61.50000000000000000, 47.04999999999999716 ) ) ;
#15550=EDGE_CURVE ( 'NONE', #11173, #5104, #3376, .T. ) ;
#15551=CARTESIAN_POINT ( 'NONE',  ( -1.035533905932738641, 66.50000000000000000, 48.35000000218494165 ) ) ;
#15552=CARTESIAN_POINT ( 'NONE',  ( 2.066987300000002303, 63.14382582708705627, 46.90000000109247225 ) ) ;
#15564=VERTEX_POINT ( 'NONE', #438 ) ;
#15574=CARTESIAN_POINT ( 'NONE',  ( -1.767766952966369765, 62.23223304703363112, 47.69999999999999574 ) ) ;
#15584=CARTESIAN_POINT ( 'NONE',  ( 4.592425496802577917E-16, 61.50000000000000000, 48.70000000218494307 ) ) ;
#15585=DIRECTION ( 'NONE',  ( -1.734723475976807094E-15, 1.000000000000000000, 0.000000000000000000 ) ) ;
#15588=FILL_AREA_STYLE_COLOUR ( '', #12558 ) ;
#15595=CARTESIAN_POINT ( 'NONE',  ( 2.066987300000002303, 63.14382582708705627, 47.50000000109246656 ) ) ;
#15596=CARTESIAN_POINT ( 'NONE',  ( -0.8561741729129461742, 66.06698730000000808, 47.20000000109246940 ) ) ;
#15612=CARTESIAN_POINT ( 'NONE',  ( 1.035533905932738197, 66.50000000000000000, 45.05000000218493739 ) ) ;
#15622=CARTESIAN_POINT ( 'NONE',  ( 0.000000000000000000, 64.00000000000000000, 49.99999999999999289 ) ) ;
#15628=( BOUNDED_CURVE ( )  B_SPLINE_CURVE ( 2, ( #13321, #105, #296, #5991, #4522, #10480, #10278, #16473, #18050 ),
 .UNSPECIFIED., .F., .F. ) 
 B_SPLINE_CURVE_WITH_KNOTS ( ( 3, 2, 2, 2, 3 ),
 ( 0.3571428571428571508, 0.3750000000000000000, 0.3928571428571427937, 0.4107142857142855874, 0.4285714285714284366 ),
 .UNSPECIFIED. ) 
 CURVE ( )  GEOMETRIC_REPRESENTATION_ITEM ( )  RATIONAL_B_SPLINE_CURVE ( ( 1.000000000000000000, 0.9238795325112867385, 1.000000000000000000, 0.9238795325112867385, 1.000000000000000000, 0.9238795325112867385, 1.000000000000000000, 0.9238795325112871826, 0.9999999999999995559 ) ) 
 REPRESENTATION_ITEM ( '' )  );
#15631=DIRECTION ( 'NONE',  ( -0.000000000000000000, -1.000000000000000000, -0.000000000000000000 ) ) ;
#15634=CARTESIAN_POINT ( 'NONE',  ( -1.530808498934192803E-16, 66.50000000000000000, 46.70000000218494307 ) ) ;
#15640=LINE ( 'NONE', #2211, #7247 ) ;
#15644=CARTESIAN_POINT ( 'NONE',  ( -1.035533905932738641, 66.50000000000000000, 49.04999999999999716 ) ) ;
#15662=CARTESIAN_POINT ( 'NONE',  ( -0.8561741729129461742, 66.06698730000000808, 45.40000000109247225 ) ) ;
#15681=CARTESIAN_POINT ( 'NONE',  ( 4.592425496802577917E-16, 61.50000000000000000, 46.30000000218493739 ) ) ;
#15693=CARTESIAN_POINT ( 'NONE',  ( -2.066987300000001415, 63.14382582708705627, 47.20000000109248361 ) ) ;
#15695=CARTESIAN_POINT ( 'NONE',  ( -1.461580736456473906, 65.46158073645646880, 48.05000000109247082 ) ) ;
#15718=CYLINDRICAL_SURFACE ( 'NONE', #6114, 2.500000000000001776 ) ;
#15738=DIRECTION ( 'NONE',  ( -0.000000000000000000, -0.000000000000000000, -1.000000000000000000 ) ) ;
#15743=CARTESIAN_POINT ( 'NONE',  ( 1.767766952966370653, 62.23223304703363112, 49.49999999999999289 ) ) ;
#15756=EDGE_CURVE ( 'NONE', #9100, #677, #3666, .T. ) ;
#15759=CARTESIAN_POINT ( 'NONE',  ( -2.066987300000001415, 64.00000000000000000, 45.55000000109246372 ) ) ;
#15763=CARTESIAN_POINT ( 'NONE',  ( 1.035533905932739751, 61.50000000000000000, 47.85000000000000142 ) ) ;
#15775=CARTESIAN_POINT ( 'NONE',  ( -2.500000000000000888, 62.96446609406726935, 46.15000000218493881 ) ) ;
#15777=EDGE_LOOP ( 'NONE', ( #6307, #13287, #1521, #9522 ) ) ;
#15785=CARTESIAN_POINT ( 'NONE',  ( 8.000000000000014211, 60.00000000000001421, 66.99999999999997158 ) ) ;
#15786=CARTESIAN_POINT ( 'NONE',  ( -1.461580736456473462, 62.53841926354353120, 45.65000000109247225 ) ) ;
#15787=CARTESIAN_POINT ( 'NONE',  ( -1.461580736456473462, 62.53841926354353120, 49.05000000109247082 ) ) ;
#15813=VERTEX_POINT ( 'NONE', #8272 ) ;
#15824=FACE_OUTER_BOUND ( 'NONE', #16105, .T. ) ;
#15833=CARTESIAN_POINT ( 'NONE',  ( -1.035533905932738641, 66.50000000000000000, 49.85000000000000142 ) ) ;
#15840=CARTESIAN_POINT ( 'NONE',  ( -7.999999999999986677, 60.00000000000000711, 45.00000000000000000 ) ) ;
#15848=CARTESIAN_POINT ( 'NONE',  ( 1.461580736456473684, 65.46158073645646880, 47.65000000109247225 ) ) ;
#15852=EDGE_CURVE ( 'NONE', #16168, #9690, #9816, .T. ) ;
#15867=CARTESIAN_POINT ( 'NONE',  ( -1.035533905932738863, 61.50000000000000000, 48.65000000218493881 ) ) ;
#15878=CARTESIAN_POINT ( 'NONE',  ( -2.066987300000001415, 63.14382582708705627, 44.80000000109247082 ) ) ;
#15913=CARTESIAN_POINT ( 'NONE',  ( -2.066987300000001415, 63.14382582708705627, 44.80000000109247082 ) ) ;
#15925=CARTESIAN_POINT ( 'NONE',  ( -2.500000000000001776, 65.03553390593273775, 49.95000000000000284 ) ) ;
#15931=CARTESIAN_POINT ( 'NONE',  ( 1.767766952966369987, 65.76776695296638309, 48.89999999999999858 ) ) ;
#15939=CARTESIAN_POINT ( 'NONE',  ( 2.066987300000001859, 63.14382582708704916, 47.50000000109246656 ) ) ;
#15943=CARTESIAN_POINT ( 'NONE',  ( -1.530808498934192803E-16, 66.50000000000000000, 49.10000000218494165 ) ) ;
#15953=VERTEX_POINT ( 'NONE', #10787 ) ;
#15961=CARTESIAN_POINT ( 'NONE',  ( -2.500000000000001776, 64.00000000000000000, 47.70000000218494307 ) ) ;
#15970=CARTESIAN_POINT ( 'NONE',  ( -1.805156233539796151, 62.95673454514856360, 44.99999999999999289 ) ) ;
#15974=CARTESIAN_POINT ( 'NONE',  ( 2.066987300000001859, 64.85617417291294373, 46.80000000109246372 ) ) ;
#15979=CARTESIAN_POINT ( 'NONE',  ( 0.9731771629430463477, 62.14345849393435373, 44.99999999999997868 ) ) ;
#16023=CYLINDRICAL_SURFACE ( 'NONE', #4032, 2.500000000000001776 ) ;
#16028=CARTESIAN_POINT ( 'NONE',  ( 2.066987300000002303, 63.14382582708705627, 46.10000000109246798 ) ) ;
#16030=( BOUNDED_CURVE ( )  B_SPLINE_CURVE ( 2, ( #9796, #6954, #18919, #11450, #19016, #7143, #19112, #4013, #5582 ),
 .UNSPECIFIED., .F., .F. ) 
 B_SPLINE_CURVE_WITH_KNOTS ( ( 3, 2, 2, 2, 3 ),
 ( 0.07142857142857121644, 0.08928571428571414892, 0.1071428571428570675, 0.1250000000000000000, 0.1428571428571429047 ),
 .UNSPECIFIED. ) 
 CURVE ( )  GEOMETRIC_REPRESENTATION_ITEM ( )  RATIONAL_B_SPLINE_CURVE ( ( 1.000000000000000666, 0.9238795325112857393, 1.000000000000000000, 0.9238795325112867385, 1.000000000000000000, 0.9238795325112867385, 1.000000000000000000, 0.9238795325112865164, 1.000000000000000222 ) ) 
 REPRESENTATION_ITEM ( '' )  );
#16041=CARTESIAN_POINT ( 'NONE',  ( -1.461580736456473462, 62.53841926354353120, 45.65000000109247225 ) ) ;
#16055=CARTESIAN_POINT ( 'NONE',  ( 1.461580736456473906, 62.53841926354353120, 48.25000000109246656 ) ) ;
#16065=ADVANCED_FACE ( 'NONE', ( #16884 ), #5302, .F. ) ;
#16066=CARTESIAN_POINT ( 'NONE',  ( 1.461580736456473684, 65.46158073645646880, 45.25000000109247367 ) ) ;
#16075=EDGE_LOOP ( 'NONE', ( #10739, #2240, #14480 ) ) ;
#16088=FACE_OUTER_BOUND ( 'NONE', #13509, .T. ) ;
#16098=PRODUCT_DEFINITION_CONTEXT ( 'detailed design', #13704, 'design' ) ;
#16105=EDGE_LOOP ( 'NONE', ( #4711, #2848, #4651, #4227 ) ) ;
#16118=CARTESIAN_POINT ( 'NONE',  ( -2.500000000000001776, 64.00000000000000000, 46.00000000000000000 ) ) ;
#16135=( BOUNDED_CURVE ( )  B_SPLINE_CURVE ( 2, ( #373, #16543, #7526, #4693, #15082, #4398, #12025, #82, #6257 ),
 .UNSPECIFIED., .F., .F. ) 
 B_SPLINE_CURVE_WITH_KNOTS ( ( 3, 2, 2, 2, 3 ),
 ( 0.2857142857142853098, 0.3035714285714282701, 0.3214285714285712858, 0.3392857142857143016, 0.3571428571428572618 ),
 .UNSPECIFIED. ) 
 CURVE ( )  GEOMETRIC_REPRESENTATION_ITEM ( )  RATIONAL_B_SPLINE_CURVE ( ( 1.000000000000001554, 0.9238795325112850731, 1.000000000000000000, 0.9238795325112867385, 1.000000000000000000, 0.9238795325112867385, 1.000000000000000000, 0.9238795325112862944, 1.000000000000000444 ) ) 
 REPRESENTATION_ITEM ( '' )  );
#16137=CARTESIAN_POINT ( 'NONE',  ( 1.461580736456473684, 65.46158073645646880, 47.85000000109246798 ) ) ;
#16152=CARTESIAN_POINT ( 'NONE',  ( -1.767766952966370209, 65.76776695296638309, 45.20000000218494307 ) ) ;
#16162=CARTESIAN_POINT ( 'NONE',  ( -2.066987300000001859, 64.85617417291294373, 44.70000000109248361 ) ) ;
#16168=VERTEX_POINT ( 'NONE', #14221 ) ;
#16184=CARTESIAN_POINT ( 'NONE',  ( 2.500000000000001776, 64.00000000000000000, 49.99999999999999289 ) ) ;
#16199=CARTESIAN_POINT ( 'NONE',  ( -1.461580736456473462, 62.53841926354353120, 44.85000000109246798 ) ) ;
#16212=CARTESIAN_POINT ( 'NONE',  ( -1.035533905932738641, 66.50000000000000000, 47.44999999999999574 ) ) ;
#16214=ORIENTED_EDGE ( 'NONE', *, *, #2551, .F. ) ;
#16217=CARTESIAN_POINT ( 'NONE',  ( -2.067357986984026397, 63.55004841362024592, 44.99999999999997868 ) ) ;
#16227=CARTESIAN_POINT ( 'NONE',  ( 8.000000000000014211, 60.00000000000000711, 45.00000000000000000 ) ) ;
#16230=CARTESIAN_POINT ( 'NONE',  ( -0.8561741729129466183, 61.93301270000000613, 48.30000000109247082 ) ) ;
#16245=CARTESIAN_POINT ( 'NONE',  ( -0.8561741729129461742, 66.06698729999999387, 48.60000000109246798 ) ) ;
#16248=CARTESIAN_POINT ( 'NONE',  ( 4.592425496802577917E-16, 61.50000000000000000, 46.19999999999999574 ) ) ;
#16255=CARTESIAN_POINT ( 'NONE',  ( -2.066987300000001415, 63.14382582708705627, 48.20000000109247651 ) ) ;
#16259=VECTOR ( 'NONE', #5093, 1000.000000000000000 ) ;
#16308=AXIS2_PLACEMENT_3D ( 'NONE', #15281, #2706, #5555 ) ;
#16315=PRODUCT ( 'Lever Press Handle Knob', 'Lever Press Handle Knob', '', ( #19137 ) ) ;
#16317=CARTESIAN_POINT ( 'NONE',  ( 1.035533905932739751, 61.50000000000000000, 47.04999999999999005 ) ) ;
#16327=VECTOR ( 'NONE', #380, 1000.000000000000000 ) ;
#16332=AXIS2_PLACEMENT_3D ( 'NONE', #10242, #8974, #2800 ) ;
#16354=CARTESIAN_POINT ( 'NONE',  ( -2.066987300000001415, 63.14382582708705627, 48.80000000109247082 ) ) ;
#16363=CARTESIAN_POINT ( 'NONE',  ( 1.461580736456473684, 65.46158073645646880, 47.85000000109246798 ) ) ;
#16365=EDGE_CURVE ( 'NONE', #17276, #3630, #19294, .T. ) ;
#16376=( BOUNDED_CURVE ( )  B_SPLINE_CURVE ( 2, ( #405, #6197, #6290, #4825, #4728, #10774, #16682, #3245, #6388 ),
 .UNSPECIFIED., .F., .F. ) 
 B_SPLINE_CURVE_WITH_KNOTS ( ( 3, 2, 2, 2, 3 ),
 ( 0.7857142857142856984, 0.8035714285714286031, 0.8214285714285713969, 0.8392857142857141906, 0.8571428571428569843 ),
 .UNSPECIFIED. ) 
 CURVE ( )  GEOMETRIC_REPRESENTATION_ITEM ( )  RATIONAL_B_SPLINE_CURVE ( ( 1.000000000000000000, 0.9238795325112867385, 1.000000000000000000, 0.9238795325112867385, 1.000000000000000000, 0.9238795325112867385, 1.000000000000000000, 0.9238795325112871826, 0.9999999999999995559 ) ) 
 REPRESENTATION_ITEM ( '' )  );
#16387=CYLINDRICAL_SURFACE ( 'NONE', #4755, 2.500000000000001776 ) ;
#16390=CARTESIAN_POINT ( 'NONE',  ( 4.592425496802577917E-16, 61.50000000000000000, 46.30000000218493739 ) ) ;
#16397=CARTESIAN_POINT ( 'NONE',  ( -1.035533905932738863, 61.50000000000000000, 47.85000000218494165 ) ) ;
#16412=CARTESIAN_POINT ( 'NONE',  ( 2.500000000000002220, 62.96446609406726935, 47.94999999999999574 ) ) ;
#16418=CARTESIAN_POINT ( 'NONE',  ( -2.152366392613727974, 63.91624855416898043, 44.99999999999999289 ) ) ;
#16435=ORIENTED_EDGE ( 'NONE', *, *, #16365, .F. ) ;
#16438=SURFACE_STYLE_FILL_AREA ( #10053 ) ;
#16448=CARTESIAN_POINT ( 'NONE',  ( -1.767766952966369765, 62.23223304703363112, 44.60000000218494165 ) ) ;
#16450=ORIENTED_EDGE ( 'NONE', *, *, #14389, .T. ) ;
#16451=CARTESIAN_POINT ( 'NONE',  ( -2.499999999999996003, 62.96446609406726225, 46.04999999999999005 ) ) ;
#16458=CARTESIAN_POINT ( 'NONE',  ( 3.796994071234847710E-16, 61.93301269999999903, 49.15000000109246514 ) ) ;
#16473=CARTESIAN_POINT ( 'NONE',  ( -2.499999999999996003, 62.96446609406726225, 46.95000000218494307 ) ) ;
#16476=AXIS2_PLACEMENT_3D ( 'NONE', #15622, #12481, #15069 ) ;
#16489=CARTESIAN_POINT ( 'NONE',  ( 2.500000000000004441, 62.96446609406726225, 46.45000000218494307 ) ) ;
#16513=CARTESIAN_POINT ( 'NONE',  ( 1.767766952966370653, 62.23223304703363112, 45.50000000000000000 ) ) ;
#16529=CARTESIAN_POINT ( 'NONE',  ( -1.909647267044692676, 63.20899822134837365, 45.00000000000000000 ) ) ;
#16543=CARTESIAN_POINT ( 'NONE',  ( -2.500000000000019096, 65.03553390593272354, 48.35000000000000853 ) ) ;
#16544=CARTESIAN_POINT ( 'NONE',  ( 0.8561741729129472844, 61.93301270000000613, 45.80000000109246372 ) ) ;
#16548=EDGE_CURVE ( 'NONE', #6405, #13224, #5266, .T. ) ;
#16550=CARTESIAN_POINT ( 'NONE',  ( -1.035533905932738863, 61.50000000000000000, 46.14999999999999858 ) ) ;
#16556=CARTESIAN_POINT ( 'NONE',  ( -2.066987300000001415, 63.14382582708705627, 49.00000000109246656 ) ) ;
#16582=DIRECTION ( 'NONE',  ( -0.000000000000000000, -0.000000000000000000, -1.000000000000000000 ) ) ;
#16652=AXIS2_PLACEMENT_3D ( 'NONE', #4874, #3490, #12309 ) ;
#16654=CARTESIAN_POINT ( 'NONE',  ( 1.461580736456473906, 62.53841926354353120, 45.85000000109246798 ) ) ;
#16660=CARTESIAN_POINT ( 'NONE',  ( -0.8561741729129461742, 66.06698730000000808, 48.60000000109246798 ) ) ;
#16662=CARTESIAN_POINT ( 'NONE',  ( 0.8561741729129472844, 61.93301270000000613, 48.40000000109247225 ) ) ;
#16664=CARTESIAN_POINT ( 'NONE',  ( 1.767766952966369987, 65.76776695296638309, 47.40000000218494591 ) ) ;
#16682=CARTESIAN_POINT ( 'NONE',  ( -1.767766952966369765, 62.23223304703363112, 45.29999999999999005 ) ) ;
#16696=CARTESIAN_POINT ( 'NONE',  ( 2.500000000000001776, 64.00000000000000000, 49.99999999999999289 ) ) ;
#16705=DIRECTION ( 'NONE',  ( 0.7071067811865463515, -0.000000000000000000, 0.7071067811865487940 ) ) ;
#16710=LINE ( 'NONE', #8084, #17519 ) ;
#16732=CARTESIAN_POINT ( 'NONE',  ( -1.752307227213768082, 62.82914575430081783, 45.02598915381526012 ) ) ;
#16733=CARTESIAN_POINT ( 'NONE',  ( -0.8561741729129461742, 66.06698729999999387, 46.40000000109246514 ) ) ;
#16743=CARTESIAN_POINT ( 'NONE',  ( 1.767766952966370653, 62.23223304703363112, 48.80000000218494449 ) ) ;
#16746=CARTESIAN_POINT ( 'NONE',  ( 0.8561741729129460632, 66.06698729999999387, 45.30000000109247082 ) ) ;
#16750=CARTESIAN_POINT ( 'NONE',  ( 2.500000000000001776, 64.00000000000000000, 45.70000000218494307 ) ) ;
#16752=VECTOR ( 'NONE', #13951, 1000.000000000000000 ) ;
#16754=DIRECTION ( 'NONE',  ( -0.7071067811865487940, 0.000000000000000000, 0.7071067811865462405 ) ) ;
#16756=CARTESIAN_POINT ( 'NONE',  ( 1.461580736456473684, 65.46158073645646880, 45.45000000109246940 ) ) ;
#16783=CARTESIAN_POINT ( 'NONE',  ( -0.8561741729129461742, 66.06698729999999387, 48.60000000109246798 ) ) ;
#16786=CARTESIAN_POINT ( 'NONE',  ( 1.035533905932739751, 61.50000000000000000, 46.35000000218494165 ) ) ;
#16808=VECTOR ( 'NONE', #2568, 1000.000000000000000 ) ;
#16810=CARTESIAN_POINT ( 'NONE',  ( -1.035533905932738641, 66.50000000000000000, 45.04999999999999005 ) ) ;
#16831=CARTESIAN_POINT ( 'NONE',  ( -1.461580736456473462, 62.53841926354353120, 48.25000000109246656 ) ) ;
#16832=LINE ( 'NONE', #13979, #14563 ) ;
#16845=CARTESIAN_POINT ( 'NONE',  ( -2.066987300000001415, 64.00000000000000000, 47.95000000109246940 ) ) ;
#16848=EDGE_CURVE ( 'NONE', #5501, #663, #12650, .T. ) ;
#16852=CARTESIAN_POINT ( 'NONE',  ( -2.066987300000001415, 64.00000000000000000, 48.75000000109246656 ) ) ;
#16854=CARTESIAN_POINT ( 'NONE',  ( 0.8561741729129472844, 61.93301270000000613, 45.20000000109248361 ) ) ;
#16856=CARTESIAN_POINT ( 'NONE',  ( 1.035533905932739751, 61.50000000000000000, 45.55000000218493739 ) ) ;
#16859=ORIENTED_EDGE ( 'NONE', *, *, #15852, .F. ) ;
#16880=CARTESIAN_POINT ( 'NONE',  ( -1.461580736456473462, 62.53841926354353120, 48.05000000109247082 ) ) ;
#16884=FACE_OUTER_BOUND ( 'NONE', #391, .T. ) ;
#16888=LINE ( 'NONE', #16696, #5224 ) ;
#16921=PLANE ( 'NONE',  #6426 ) ;
#16931=CARTESIAN_POINT ( 'NONE',  ( -1.265664690411616068E-16, 66.06698730000000808, 48.75000000109246656 ) ) ;
#16947=CARTESIAN_POINT ( 'NONE',  ( -2.066987300000001859, 64.85617417291294373, 47.10000000109246798 ) ) ;
#16953=DIRECTION ( 'NONE',  ( 0.000000000000000000, 1.000000000000000000, 0.000000000000000000 ) ) ;
#16956=CARTESIAN_POINT ( 'NONE',  ( 2.066987300000001859, 64.85617417291294373, 45.40000000109246514 ) ) ;
#16976=ORIENTED_EDGE ( 'NONE', *, *, #11313, .F. ) ;
#16985=CARTESIAN_POINT ( 'NONE',  ( -2.066987300000001415, 63.14382582708705627, 48.00000000109246656 ) ) ;
#16988=DIRECTION ( 'NONE',  ( -0.000000000000000000, -0.000000000000000000, -1.000000000000000000 ) ) ;
#16992=ORIENTED_EDGE ( 'NONE', *, *, #847, .F. ) ;
#17001=VERTEX_POINT ( 'NONE', #1004 ) ;
#17029=CARTESIAN_POINT ( 'NONE',  ( 2.066987300000001415, 64.00000000000000000, 46.95000000109246940 ) ) ;
#17047=DIRECTION ( 'NONE',  ( -0.000000000000000000, -0.000000000000000000, -1.000000000000000000 ) ) ;
#17062=CARTESIAN_POINT ( 'NONE',  ( 2.500000000000002220, 62.96446609406726935, 46.45000000218495018 ) ) ;
#17063=CARTESIAN_POINT ( 'NONE',  ( 8.000000000000014211, 60.00000000000000711, 45.00000000000000000 ) ) ;
#17067=( NAMED_UNIT ( * ) PLANE_ANGLE_UNIT ( ) SI_UNIT ( $, .RADIAN. ) );
#17075=CARTESIAN_POINT ( 'NONE',  ( 2.066987300000001859, 64.85617417291294373, 47.60000000109246798 ) ) ;
#17076=CARTESIAN_POINT ( 'NONE',  ( 1.461580736456473684, 65.46158073645646880, 48.65000000109247225 ) ) ;
#17095=LINE ( 'NONE', #17186, #16752 ) ;
#17098=CARTESIAN_POINT ( 'NONE',  ( -1.530808498934192803E-16, 66.50000000000000000, 46.59999999999999432 ) ) ;
#17110=DIRECTION ( 'NONE',  ( 0.000000000000000000, 1.000000000000000000, 0.000000000000000000 ) ) ;
#17113=CARTESIAN_POINT ( 'NONE',  ( -2.500000000000001776, 64.00000000000000000, 46.79999999999999716 ) ) ;
#17120=CARTESIAN_POINT ( 'NONE',  ( -2.066987300000001415, 64.00000000000000000, 48.15000000109247225 ) ) ;
#17135=CARTESIAN_POINT ( 'NONE',  ( 3.796994071234847710E-16, 61.93301269999999903, 47.35000000109246798 ) ) ;
#17138=CARTESIAN_POINT ( 'NONE',  ( -1.461580736456473462, 62.53841926354353120, 45.05000000109246372 ) ) ;
#17153=CARTESIAN_POINT ( 'NONE',  ( -2.500000000000001776, 65.03553390593273775, 46.85000000218494165 ) ) ;
#17166=CARTESIAN_POINT ( 'NONE',  ( -0.8561741729129465073, 61.93301270000000613, 47.30000000109247082 ) ) ;
#17167=CARTESIAN_POINT ( 'NONE',  ( 0.8561741729129460632, 66.06698730000000808, 49.50000000109246656 ) ) ;
#17176=ORIENTED_EDGE ( 'NONE', *, *, #12727, .F. ) ;
#17186=CARTESIAN_POINT ( 'NONE',  ( 2.500000000000001776, 64.00000000000000000, 49.99999999999999289 ) ) ;
#17208=CARTESIAN_POINT ( 'NONE',  ( -1.035533905932738641, 66.50000000000000000, 46.75000000218494733 ) ) ;
#17216=CARTESIAN_POINT ( 'NONE',  ( -2.066987300000001415, 64.00000000000000000, 44.95000000109246940 ) ) ;
#17222=CARTESIAN_POINT ( 'NONE',  ( -1.035533905932738641, 66.50000000000000000, 49.04999999999999716 ) ) ;
#17227=LINE ( 'NONE', #11326, #2200 ) ;
#17231=CARTESIAN_POINT ( 'NONE',  ( 2.066987300000001415, 64.85617417291294373, 46.80000000109247082 ) ) ;
#17246=CARTESIAN_POINT ( 'NONE',  ( 1.767766952966370653, 62.23223304703363112, 46.40000000218494591 ) ) ;
#17258=CARTESIAN_POINT ( 'NONE',  ( -2.066987300000001415, 64.00000000000000000, 45.55000000109246372 ) ) ;
#17260=CARTESIAN_POINT ( 'NONE',  ( -2.066987300000001415, 64.00000000000000000, 48.15000000109247225 ) ) ;
#17276=VERTEX_POINT ( 'NONE', #4933 ) ;
#17279=ORIENTED_EDGE ( 'NONE', *, *, #14860, .T. ) ;
#17283=CARTESIAN_POINT ( 'NONE',  ( 2.500000000000001776, 64.00000000000000000, 49.99999999999999289 ) ) ;
#17290=( BOUNDED_CURVE ( )  B_SPLINE_CURVE ( 2, ( #11953, #10273, #8712, #9110, #5882 ),
 .UNSPECIFIED., .F., .F. ) 
 B_SPLINE_CURVE_WITH_KNOTS ( ( 3, 2, 3 ),
 ( 0.8571428571428569843, 0.8750000000000000000, 0.8928571428571429047 ),
 .UNSPECIFIED. ) 
 CURVE ( )  GEOMETRIC_REPRESENTATION_ITEM ( )  RATIONAL_B_SPLINE_CURVE ( ( 1.000000000000000444, 0.9238795325112862944, 1.000000000000000000, 0.9238795325112867385, 1.000000000000000000 ) ) 
 REPRESENTATION_ITEM ( '' )  );
#17308=CARTESIAN_POINT ( 'NONE',  ( -1.767766952966369765, 62.23223304703363112, 49.29999999999999716 ) ) ;
#17336=CARTESIAN_POINT ( 'NONE',  ( 1.035533905932739751, 61.50000000000000000, 47.15000000218494591 ) ) ;
#17347=CARTESIAN_POINT ( 'NONE',  ( 0.8561741729129460632, 66.06698729999999387, 45.30000000109247082 ) ) ;
#17367=LINE ( 'NONE', #17283, #7885 ) ;
#17396=CARTESIAN_POINT ( 'NONE',  ( -0.8561741729129465073, 61.93301270000000613, 45.90000000109247225 ) ) ;
#17403=CARTESIAN_POINT ( 'NONE',  ( -2.500000000000001776, 64.00000000000000000, 49.19999999999999574 ) ) ;
#17408=EDGE_CURVE ( 'NONE', #1259, #14616, #13946, .T. ) ;
#17411=CARTESIAN_POINT ( 'NONE',  ( 2.066987300000001415, 64.85617417291294373, 47.60000000109246798 ) ) ;
#17430=CARTESIAN_POINT ( 'NONE',  ( 2.500000000000001776, 65.03553390593273775, 47.35000000218494165 ) ) ;
#17437=CARTESIAN_POINT ( 'NONE',  ( -1.038177767593160716, 62.20757355991266024, 44.99999999999999289 ) ) ;
#17440=CARTESIAN_POINT ( 'NONE',  ( 1.461580736456473684, 65.46158073645646880, 46.85000000109246798 ) ) ;
#17476=FACE_OUTER_BOUND ( 'NONE', #9408, .T. ) ;
#17484=CARTESIAN_POINT ( 'NONE',  ( -1.265664690411616068E-16, 66.06698730000000808, 44.75000000109247367 ) ) ;
#17489=EDGE_CURVE ( 'NONE', #15813, #677, #879, .T. ) ;
#17501=CARTESIAN_POINT ( 'NONE',  ( -0.8561741729129461742, 66.06698730000000808, 47.00000000109247367 ) ) ;
#17503=( BOUNDED_SURFACE ( )  B_SPLINE_SURFACE ( 1, 2, ( 
 ( #9079, #15066, #162, #2904, #6148, #12108, #18105, #7916, #15354, #4788, #3586, #12602, #1829, #5072, #15453, #14075, #8012, #13978, #1933, #12408, #16931, #18502, #4972, #6243, #5161, #13879, #7809, #10836, #12502, #647, #16831, #9272, #17120, #3392, #455, #11124, #3303, #18307, #9559, #10929, #6441, #10737, #9467, #3684, #9363, #18406, #3493, #257, #2020, #9653, #13781, #11027, #550, #6637, #6536, #18594, #17029, #15552, #2121, #4876, #8105, #1732, #15258, #7712, #13678, #12209, #18210, #16733, #360, #6347, #12312, #741, #11496, #16028, #14351, #2588, #5257, #17396, #6814, #2489, #10027, #11399, #4169, #9836, #3870, #5633, #9752, #1120, #18881, #11209, #11595, #5351, #8477, #7002, #5538, #19060, #17216, #8206, #17592, #3783, #17484 ),
 ( #5444, #15925, #4062, #15833, #11314, #2396, #3969, #8381, #6719, #926, #15743, #2305, #6909, #18969, #17308, #9927, #12881, #8569, #14454, #15644, #14548, #1028, #12970, #7099, #12691, #13064, #2214, #14172, #18693, #8289, #14261, #832, #12780, #18778, #13168, #11990, #1621, #10225, #13463, #4465, #3075, #16412, #2976, #4362, #1417, #5926, #7487, #13365, #14644, #13559, #2882, #16212, #19260, #1519, #9055, #5832, #17685, #6121, #11795, #16317, #140, #11693, #7295, #17983, #19357, #8860, #19163, #17892, #12088, #17788, #10319, #14845, #8664, #7394, #18084, #2780, #45, #8957, #13261, #6030, #16118, #15042, #4559, #10416, #4265, #11895, #14946, #10517, #8758, #1213, #16513, #5734, #7593, #10120, #2688, #7193, #14747, #1323, #623, #16810, #3473 ) ),
 .UNSPECIFIED., .F., .F., .F. ) 
 B_SPLINE_SURFACE_WITH_KNOTS ( ( 2, 2 ),
 ( 3, 2, 2, 2, 2, 2, 2, 2, 2, 2, 2, 2, 2, 2, 2, 2, 2, 2, 2, 2, 2, 2, 2, 2, 2, 2, 2, 2, 2, 2, 2, 2, 2, 2, 2, 2, 2, 2, 2, 2, 2, 2, 2, 2, 2, 2, 2, 2, 2, 2, 3 ),
 ( 0.000000000000000000, 1.000000000000000000 ),
 ( 0.000000000000000000, 0.01785714285714285615, 0.03571428571428571230, 0.05357142857142856845, 0.07142857142857142461, 0.08928571428571428770, 0.1071428571428571369, 0.1250000000000000000, 0.1428571428571428492, 0.1607142857142857262, 0.1785714285714285754, 0.1964285714285714246, 0.2142857142857142738, 0.2321428571428571508, 0.2500000000000000000, 0.2678571428571428492, 0.2857142857142856984, 0.3035714285714285476, 0.3214285714285714524, 0.3392857142857143016, 0.3571428571428571508, 0.3750000000000000000, 0.3928571428571428492, 0.4107142857142856984, 0.4285714285714285476, 0.4464285714285714524, 0.4642857142857143016, 0.4821428571428571508, 0.5000000000000000000, 0.5178571428571429047, 0.5357142857142856984, 0.5535714285714286031, 0.5714285714285713969, 0.5892857142857143016, 0.6071428571428570953, 0.6250000000000000000, 0.6428571428571429047, 0.6607142857142856984, 0.6785714285714286031, 0.6964285714285713969, 0.7142857142857143016, 0.7321428571428570953, 0.7500000000000000000, 0.7678571428571429047, 0.7857142857142856984, 0.8035714285714286031, 0.8214285714285713969, 0.8392857142857143016, 0.8571428571428570953, 0.8750000000000000000, 0.8928571428571429047 ),
 .UNSPECIFIED. ) 
 GEOMETRIC_REPRESENTATION_ITEM ( )  RATIONAL_B_SPLINE_SURFACE ( (
 ( 1.000000000000000000, 0.9238795325112867385, 1.000000000000000000, 0.9238795325112867385, 1.000000000000000000, 0.9238795325112867385, 1.000000000000000000, 0.9238795325112867385, 1.000000000000000000, 0.9238795325112867385, 1.000000000000000000, 0.9238795325112867385, 1.000000000000000000, 0.9238795325112867385, 1.000000000000000000, 0.9238795325112867385, 1.000000000000000000, 0.9238795325112867385, 1.000000000000000000, 0.9238795325112867385, 1.000000000000000000, 0.9238795325112867385, 1.000000000000000000, 0.9238795325112867385, 1.000000000000000000, 0.9238795325112867385, 1.000000000000000000, 0.9238795325112867385, 1.000000000000000000, 0.9238795325112867385, 1.000000000000000000, 0.9238795325112867385, 1.000000000000000000, 0.9238795325112867385, 1.000000000000000000, 0.9238795325112867385, 1.000000000000000000, 0.9238795325112867385, 1.000000000000000000, 0.9238795325112867385, 1.000000000000000000, 0.9238795325112867385, 1.000000000000000000, 0.9238795325112867385, 1.000000000000000000, 0.9238795325112867385, 1.000000000000000000, 0.9238795325112867385, 1.000000000000000000, 0.9238795325112867385, 1.000000000000000000, 0.9238795325112867385, 1.000000000000000000, 0.9238795325112867385, 1.000000000000000000, 0.9238795325112867385, 1.000000000000000000, 0.9238795325112867385, 1.000000000000000000, 0.9238795325112867385, 1.000000000000000000, 0.9238795325112867385, 1.000000000000000000, 0.9238795325112867385, 1.000000000000000000, 0.9238795325112867385, 1.000000000000000000, 0.9238795325112867385, 1.000000000000000000, 0.9238795325112867385, 1.000000000000000000, 0.9238795325112867385, 1.000000000000000000, 0.9238795325112867385, 1.000000000000000000, 0.9238795325112867385, 1.000000000000000000, 0.9238795325112867385, 1.000000000000000000, 0.9238795325112867385, 1.000000000000000000, 0.9238795325112867385, 1.000000000000000000, 0.9238795325112867385, 1.000000000000000000, 0.9238795325112867385, 1.000000000000000000, 0.9238795325112867385, 1.000000000000000000, 0.9238795325112867385, 1.000000000000000000, 0.9238795325112867385, 1.000000000000000000, 0.9238795325112867385, 1.000000000000000000, 0.9238795325112867385, 1.000000000000000000, 0.9238795325112867385, 1.000000000000000000, 0.9238795325112867385, 1.000000000000000000),
 ( 1.000000000000000000, 0.9238795325112867385, 1.000000000000000000, 0.9238795325112867385, 1.000000000000000000, 0.9238795325112867385, 1.000000000000000000, 0.9238795325112867385, 1.000000000000000000, 0.9238795325112867385, 1.000000000000000000, 0.9238795325112867385, 1.000000000000000000, 0.9238795325112867385, 1.000000000000000000, 0.9238795325112867385, 1.000000000000000000, 0.9238795325112867385, 1.000000000000000000, 0.9238795325112867385, 1.000000000000000000, 0.9238795325112867385, 1.000000000000000000, 0.9238795325112867385, 1.000000000000000000, 0.9238795325112867385, 1.000000000000000000, 0.9238795325112867385, 1.000000000000000000, 0.9238795325112867385, 1.000000000000000000, 0.9238795325112867385, 1.000000000000000000, 0.9238795325112867385, 1.000000000000000000, 0.9238795325112867385, 1.000000000000000000, 0.9238795325112867385, 1.000000000000000000, 0.9238795325112867385, 1.000000000000000000, 0.9238795325112867385, 1.000000000000000000, 0.9238795325112867385, 1.000000000000000000, 0.9238795325112867385, 1.000000000000000000, 0.9238795325112867385, 1.000000000000000000, 0.9238795325112867385, 1.000000000000000000, 0.9238795325112867385, 1.000000000000000000, 0.9238795325112867385, 1.000000000000000000, 0.9238795325112867385, 1.000000000000000000, 0.9238795325112867385, 1.000000000000000000, 0.9238795325112867385, 1.000000000000000000, 0.9238795325112867385, 1.000000000000000000, 0.9238795325112867385, 1.000000000000000000, 0.9238795325112867385, 1.000000000000000000, 0.9238795325112867385, 1.000000000000000000, 0.9238795325112867385, 1.000000000000000000, 0.9238795325112867385, 1.000000000000000000, 0.9238795325112867385, 1.000000000000000000, 0.9238795325112867385, 1.000000000000000000, 0.9238795325112867385, 1.000000000000000000, 0.9238795325112867385, 1.000000000000000000, 0.9238795325112867385, 1.000000000000000000, 0.9238795325112867385, 1.000000000000000000, 0.9238795325112867385, 1.000000000000000000, 0.9238795325112867385, 1.000000000000000000, 0.9238795325112867385, 1.000000000000000000, 0.9238795325112867385, 1.000000000000000000, 0.9238795325112867385, 1.000000000000000000, 0.9238795325112867385, 1.000000000000000000, 0.9238795325112867385, 1.000000000000000000, 0.9238795325112867385, 1.000000000000000000) ) ) 
 REPRESENTATION_ITEM ( '' )  SURFACE ( )  );
#17505=DIRECTION ( 'NONE',  ( 0.000000000000000000, 0.000000000000000000, -1.000000000000000000 ) ) ;
#17515=VERTEX_POINT ( 'NONE', #3642 ) ;
#17519=VECTOR ( 'NONE', #10808, 1000.000000000000000 ) ;
#17521=CARTESIAN_POINT ( 'NONE',  ( -1.461580736456473906, 65.46158073645646880, 48.65000000109247225 ) ) ;
#17522=CARTESIAN_POINT ( 'NONE',  ( 8.000000000000000000, 68.00000000000000000, 45.00000000000000000 ) ) ;
#17536=CARTESIAN_POINT ( 'NONE',  ( 1.461580736456473906, 62.53841926354353120, 45.05000000109246372 ) ) ;
#17587=CARTESIAN_POINT ( 'NONE',  ( -2.500000000000006661, 65.03553390593272354, 46.85000000218494165 ) ) ;
#17592=CARTESIAN_POINT ( 'NONE',  ( -1.461580736456473906, 65.46158073645646880, 44.85000000109246798 ) ) ;
#17595=ORIENTED_EDGE ( 'NONE', *, *, #17939, .F. ) ;
#17608=CARTESIAN_POINT ( 'NONE',  ( 2.066987300000001415, 64.85617417291294373, 47.00000000109246656 ) ) ;
#17615=CARTESIAN_POINT ( 'NONE',  ( -1.035533905932738641, 66.50000000000000000, 47.44999999999998863 ) ) ;
#17621=CARTESIAN_POINT ( 'NONE',  ( -2.066987300000001415, 64.00000000000000000, 48.75000000109246656 ) ) ;
#17627=CARTESIAN_POINT ( 'NONE',  ( -1.767766952966369765, 62.23223304703363112, 46.09999999999999432 ) ) ;
#17633=CARTESIAN_POINT ( 'NONE',  ( 2.066987300000001415, 64.00000000000000000, 49.35000000109246798 ) ) ;
#17643=EDGE_CURVE ( 'NONE', #17922, #9572, #12675, .T. ) ;
#17685=CARTESIAN_POINT ( 'NONE',  ( 2.500000000000001776, 64.00000000000000000, 47.19999999999999574 ) ) ;
#17687=PRODUCT_DEFINITION_FORMATION_WITH_SPECIFIED_SOURCE ( 'ANY', '', #16315, .NOT_KNOWN. ) ;
#17703=LINE ( 'NONE', #13187, #5379 ) ;
#17704=CARTESIAN_POINT ( 'NONE',  ( 2.066987300000001859, 63.14382582708704916, 48.50000000109246656 ) ) ;
#17720=CARTESIAN_POINT ( 'NONE',  ( -2.500000000000001776, 64.00000000000000000, 45.30000000218493739 ) ) ;
#17721=CARTESIAN_POINT ( 'NONE',  ( 2.500000000000002220, 62.96446609406726935, 44.85000000218494165 ) ) ;
#17731=CARTESIAN_POINT ( 'NONE',  ( 0.8561741729129472844, 61.93301270000000613, 46.00000000109245946 ) ) ;
#17788=CARTESIAN_POINT ( 'NONE',  ( 1.035533905932738197, 66.50000000000000000, 46.54999999999999716 ) ) ;
#17807=CARTESIAN_POINT ( 'NONE',  ( 2.066987300000001415, 64.85617417291294373, 45.40000000109247225 ) ) ;
#17822=CARTESIAN_POINT ( 'NONE',  ( -1.767766952966370209, 65.76776695296638309, 46.00000000218494733 ) ) ;
#17832=CARTESIAN_POINT ( 'NONE',  ( -2.066987300000001415, 64.00000000000000000, 48.15000000109247225 ) ) ;
#17851=EDGE_CURVE ( 'NONE', #14201, #11173, #10519, .T. ) ;
#17855=DIRECTION ( 'NONE',  ( 0.000000000000000000, 0.000000000000000000, 1.000000000000000000 ) ) ;
#17872=EDGE_CURVE ( 'NONE', #15564, #18046, #1897, .T. ) ;
#17874=CARTESIAN_POINT ( 'NONE',  ( 1.767766952966370653, 62.23223304703363112, 48.00000000218494023 ) ) ;
#17892=CARTESIAN_POINT ( 'NONE',  ( -1.035533905932738641, 66.50000000000000000, 46.64999999999999147 ) ) ;
#17900=CARTESIAN_POINT ( 'NONE',  ( -2.000850093858623779, 63.37525195204790407, 45.00000000000001421 ) ) ;
#17913=CARTESIAN_POINT ( 'NONE',  ( -0.8561741729129466183, 61.93301270000000613, 45.10000000109246798 ) ) ;
#17922=VERTEX_POINT ( 'NONE', #12800 ) ;
#17927=CARTESIAN_POINT ( 'NONE',  ( 4.592425496802577917E-16, 61.50000000000000000, 45.50000000218494733 ) ) ;
#17930=CARTESIAN_POINT ( 'NONE',  ( 1.767766952966370653, 62.23223304703363112, 46.29999999999999716 ) ) ;
#17936=CARTESIAN_POINT ( 'NONE',  ( 2.066987300000001415, 64.00000000000000000, 46.95000000109246940 ) ) ;
#17937=DIRECTION ( 'NONE',  ( -1.000000000000000000, 0.000000000000000000, -0.000000000000000000 ) ) ;
#17939=EDGE_CURVE ( 'NONE', #2362, #6663, #10631, .T. ) ;
#17951=ORIENTED_EDGE ( 'NONE', *, *, #8125, .F. ) ;
#17954=ORIENTED_EDGE ( 'NONE', *, *, #16548, .F. ) ;
#17969=CARTESIAN_POINT ( 'NONE',  ( 4.592425496802577917E-16, 61.50000000000000000, 47.90000000218494591 ) ) ;
#17983=CARTESIAN_POINT ( 'NONE',  ( -2.500000000000000888, 62.96446609406726935, 46.84999999999998721 ) ) ;
#18007=CARTESIAN_POINT ( 'NONE',  ( -2.066987300000001415, 64.85617417291294373, 46.50000000109246656 ) ) ;
#18024=CARTESIAN_POINT ( 'NONE',  ( -0.8561741729129465073, 61.93301270000000613, 48.10000000109246798 ) ) ;
#18032=CARTESIAN_POINT ( 'NONE',  ( -0.8561741729129461742, 66.06698729999999387, 46.40000000109246514 ) ) ;
#18044=( BOUNDED_CURVE ( )  B_SPLINE_CURVE ( 2, ( #3109, #13498, #16743, #19292, #4496, #10552, #3011, #9188, #8988 ),
 .UNSPECIFIED., .F., .F. ) 
 B_SPLINE_CURVE_WITH_KNOTS ( ( 3, 2, 2, 2, 3 ),
 ( 0.07142857142857156338, 0.08928571428571438484, 0.1071428571428571924, 0.1250000000000000000, 0.1428571428571428215 ),
 .UNSPECIFIED. ) 
 CURVE ( )  GEOMETRIC_REPRESENTATION_ITEM ( )  RATIONAL_B_SPLINE_CURVE ( ( 0.9999999999999994449, 0.9238795325112872936, 1.000000000000000000, 0.9238795325112867385, 1.000000000000000000, 0.9238795325112867385, 1.000000000000000000, 0.9238795325112868495, 0.9999999999999998890 ) ) 
 REPRESENTATION_ITEM ( '' )  );
#18046=VERTEX_POINT ( 'NONE', #5184 ) ;
#18050=CARTESIAN_POINT ( 'NONE',  ( -2.500000000000001776, 64.00000000000000000, 46.90000000218494591 ) ) ;
#18073=CYLINDRICAL_SURFACE ( 'NONE', #4451, 2.500000000000001776 ) ;
#18084=CARTESIAN_POINT ( 'NONE',  ( 1.767766952966370653, 62.23223304703363112, 46.29999999999999716 ) ) ;
#18103=CARTESIAN_POINT ( 'NONE',  ( -2.500000000000001776, 64.00000000000000000, 49.19999999999999574 ) ) ;
#18104=CARTESIAN_POINT ( 'NONE',  ( -1.265664690411616068E-16, 66.06698730000000808, 46.35000000109246798 ) ) ;
#18105=CARTESIAN_POINT ( 'NONE',  ( 1.461580736456473684, 65.46158073645646880, 49.45000000109246940 ) ) ;
#18120=CARTESIAN_POINT ( 'NONE',  ( 2.066987300000002303, 63.14382582708705627, 45.90000000109247225 ) ) ;
#18126=CARTESIAN_POINT ( 'NONE',  ( -2.066987300000000971, 63.14382582708704916, 48.80000000109247082 ) ) ;
#18129=CARTESIAN_POINT ( 'NONE',  ( -1.265664690411616068E-16, 66.06698730000000808, 46.35000000109246798 ) ) ;
#18187=DIRECTION ( 'NONE',  ( 0.000000000000000000, 0.000000000000000000, 1.000000000000000000 ) ) ;
#18203=CARTESIAN_POINT ( 'NONE',  ( 2.500000000000001776, 64.00000000000000000, 47.19999999999999574 ) ) ;
#18208=CYLINDRICAL_SURFACE ( 'NONE', #10999, 2.500000000000001776 ) ;
#18210=CARTESIAN_POINT ( 'NONE',  ( -1.461580736456473906, 65.46158073645646880, 46.45000000109246940 ) ) ;
#18224=CARTESIAN_POINT ( 'NONE',  ( -1.461580736456473462, 62.53841926354353120, 46.45000000109246940 ) ) ;
#18231=CARTESIAN_POINT ( 'NONE',  ( 0.8561741729129471734, 61.93301270000000613, 48.20000000109247651 ) ) ;
#18233=CARTESIAN_POINT ( 'NONE',  ( -1.461580736456473462, 62.53841926354353120, 45.85000000109246798 ) ) ;
#18235=CARTESIAN_POINT ( 'NONE',  ( 4.592425496802577917E-16, 61.50000000000000000, 45.50000000218494733 ) ) ;
#18253=EDGE_CURVE ( 'NONE', #1259, #17515, #13968, .T. ) ;
#18268=ORIENTED_EDGE ( 'NONE', *, *, #10546, .T. ) ;
#18271=ADVANCED_FACE ( 'NONE', ( #1645 ), #4680, .F. ) ;
#18307=CARTESIAN_POINT ( 'NONE',  ( 0.8561741729129460632, 66.06698729999999387, 47.90000000109247225 ) ) ;
#18320=CARTESIAN_POINT ( 'NONE',  ( 2.066987300000001415, 64.00000000000000000, 45.15000000109247225 ) ) ;
#18321=ORIENTED_EDGE ( 'NONE', *, *, #8403, .T. ) ;
#18337=VERTEX_POINT ( 'NONE', #13812 ) ;
#18351=LINE ( 'NONE', #10881, #5043 ) ;
#18356=CARTESIAN_POINT ( 'NONE',  ( -0.8561741729129461742, 66.06698729999999387, 47.80000000109247082 ) ) ;
#18392=( BOUNDED_CURVE ( )  B_SPLINE_CURVE ( 2, ( #9922, #17587, #14346, #17208, #15634, #6809, #3774, #2482, #2300 ),
 .UNSPECIFIED., .F., .F. ) 
 B_SPLINE_CURVE_WITH_KNOTS ( ( 3, 2, 2, 2, 3 ),
 ( 0.4285714285714284366, 0.4464285714285713413, 0.4642857142857141906, 0.4821428571428570953, 0.4999999999999999445 ),
 .UNSPECIFIED. ) 
 CURVE ( )  GEOMETRIC_REPRESENTATION_ITEM ( )  RATIONAL_B_SPLINE_CURVE ( ( 1.000000000000000444, 0.9238795325112862944, 1.000000000000000000, 0.9238795325112867385, 1.000000000000000000, 0.9238795325112867385, 1.000000000000000000, 0.9238795325112869605, 0.9999999999999997780 ) ) 
 REPRESENTATION_ITEM ( '' )  );
#18406=CARTESIAN_POINT ( 'NONE',  ( -0.8561741729129465073, 61.93301270000000613, 47.50000000109246656 ) ) ;
#18420=CARTESIAN_POINT ( 'NONE',  ( -0.8561741729129465073, 61.93301270000000613, 45.70000000109248361 ) ) ;
#18423=CARTESIAN_POINT ( 'NONE',  ( -1.767766952966370209, 65.76776695296638309, 46.00000000218494733 ) ) ;
#18429=CARTESIAN_POINT ( 'NONE',  ( -2.499999999999992450, 65.03553390593275196, 47.65000000218494591 ) ) ;
#18449=DIRECTION ( 'NONE',  ( 1.734723475976807094E-15, -1.000000000000000000, 0.000000000000000000 ) ) ;
#18451=FACE_OUTER_BOUND ( 'NONE', #9341, .T. ) ;
#18477=CARTESIAN_POINT ( 'NONE',  ( 2.500000000000001776, 64.00000000000000000, 46.39999999999999858 ) ) ;
#18500=FACE_OUTER_BOUND ( 'NONE', #15777, .T. ) ;
#18502=CARTESIAN_POINT ( 'NONE',  ( 0.8561741729129460632, 66.06698729999999387, 48.70000000109247651 ) ) ;
#18516=STYLED_ITEM ( 'NONE', ( #2156 ), #3958 ) ;
#18524=CARTESIAN_POINT ( 'NONE',  ( -1.461580736456473462, 62.53841926354353120, 48.05000000109247082 ) ) ;
#18526=AXIS2_PLACEMENT_3D ( 'NONE', #4657, #18187, #3180 ) ;
#18558=CARTESIAN_POINT ( 'NONE',  ( 1.461580736456473906, 62.53841926354353120, 47.65000000109247225 ) ) ;
#18594=CARTESIAN_POINT ( 'NONE',  ( 2.066987300000001859, 64.85617417291294373, 47.00000000109246656 ) ) ;
#18596=EDGE_CURVE ( 'NONE', #17276, #14706, #12859, .T. ) ;
#18612=CARTESIAN_POINT ( 'NONE',  ( -2.066987300000001415, 64.85617417291294373, 46.30000000109247082 ) ) ;
#18631=CARTESIAN_POINT ( 'NONE',  ( -1.767766952966369765, 62.23223304703363112, 47.80000000218494449 ) ) ;
#18645=CARTESIAN_POINT ( 'NONE',  ( 0.8561741729129472844, 61.93301270000000613, 47.40000000109247225 ) ) ;
#18647=CARTESIAN_POINT ( 'NONE',  ( 1.461580736456473906, 62.53841926354353120, 46.85000000109246798 ) ) ;
#18648=CYLINDRICAL_SURFACE ( 'NONE', #7205, 2.500000000000001776 ) ;
#18652=CARTESIAN_POINT ( 'NONE',  ( 1.466517438298505116, 62.42153833278998576, 44.99999999999999289 ) ) ;
#18693=CARTESIAN_POINT ( 'NONE',  ( 4.592425496802577917E-16, 61.50000000000000000, 48.59999999999999432 ) ) ;
#18694=CARTESIAN_POINT ( 'NONE',  ( -7.999999999999986677, 68.00000000000000000, 45.00000000000000000 ) ) ;
#18706=CARTESIAN_POINT ( 'NONE',  ( -1.461580736456473462, 62.53841926354353120, 46.45000000109246940 ) ) ;
#18709=LINE ( 'NONE', #9945, #8779 ) ;
#18720=CARTESIAN_POINT ( 'NONE',  ( 1.035533905932739751, 61.50000000000000000, 47.95000000218495018 ) ) ;
#18733=CARTESIAN_POINT ( 'NONE',  ( -0.8561741729129465073, 61.93301270000000613, 46.50000000109247367 ) ) ;
#18734=CARTESIAN_POINT ( 'NONE',  ( 3.796994071234847710E-16, 61.93301269999999903, 47.55000000109247082 ) ) ;
#18767=DIRECTION ( 'NONE',  ( -1.000000000000000000, 0.000000000000000000, -0.000000000000000000 ) ) ;
#18778=CARTESIAN_POINT ( 'NONE',  ( -2.500000000000001776, 65.03553390593273775, 48.35000000000000142 ) ) ;
#18793=CARTESIAN_POINT ( 'NONE',  ( 0.8561741729129460632, 66.06698730000000808, 45.30000000109246372 ) ) ;
#18800=CARTESIAN_POINT ( 'NONE',  ( 2.499999999999996891, 62.96446609406726225, 47.94999999999998863 ) ) ;
#18813=CARTESIAN_POINT ( 'NONE',  ( 1.767766952966370653, 62.23223304703363112, 48.00000000218494023 ) ) ;
#18814=CARTESIAN_POINT ( 'NONE',  ( -2.500000000000001776, 64.00000000000000000, 49.30000000218494449 ) ) ;
#18824=CARTESIAN_POINT ( 'NONE',  ( -2.066987300000001859, 64.85617417291294373, 45.50000000109247367 ) ) ;
#18845=ORIENTED_EDGE ( 'NONE', *, *, #6958, .T. ) ;
#18855=EDGE_CURVE ( 'NONE', #13224, #2362, #16888, .T. ) ;
#18881=CARTESIAN_POINT ( 'NONE',  ( 2.066987300000001415, 64.00000000000000000, 45.35000000109246798 ) ) ;
#18887=CARTESIAN_POINT ( 'NONE',  ( 2.499999999999996003, 65.03553390593275196, 48.85000000000000142 ) ) ;
#18894=CARTESIAN_POINT ( 'NONE',  ( -0.8561741729129466183, 61.93301270000000613, 46.50000000109247367 ) ) ;
#18907=CARTESIAN_POINT ( 'NONE',  ( -1.530808498934192803E-16, 66.50000000000000000, 47.50000000218494023 ) ) ;
#18917=CARTESIAN_POINT ( 'NONE',  ( 2.066987300000002303, 63.14382582708705627, 49.30000000109246372 ) ) ;
#18919=CARTESIAN_POINT ( 'NONE',  ( 1.767766952966370653, 62.23223304703363112, 49.49999999999999289 ) ) ;
#18955=ORIENTED_EDGE ( 'NONE', *, *, #8403, .F. ) ;
#18969=CARTESIAN_POINT ( 'NONE',  ( -1.035533905932738863, 61.50000000000000000, 49.35000000000000142 ) ) ;
#18984=CARTESIAN_POINT ( 'NONE',  ( 0.8561741729129460632, 66.06698730000000808, 46.90000000109247225 ) ) ;
#19003=CARTESIAN_POINT ( 'NONE',  ( 2.500000000000001776, 65.03553390593273775, 46.55000000218494449 ) ) ;
#19011=CARTESIAN_POINT ( 'NONE',  ( 0.7910017786515960436, 62.09035273295529578, 44.99999999999998579 ) ) ;
#19014=CARTESIAN_POINT ( 'NONE',  ( -0.8561741729129461742, 66.06698729999999387, 46.20000000109247651 ) ) ;
#19016=CARTESIAN_POINT ( 'NONE',  ( 4.592425496802577917E-16, 61.50000000000000000, 49.39999999999999147 ) ) ;
#19047=AXIS2_PLACEMENT_3D ( 'NONE', #5348, #19057, #12778 ) ;
#19048=CARTESIAN_POINT ( 'NONE',  ( 2.500000000000001776, 64.00000000000000000, 48.79999999999999716 ) ) ;
#19057=DIRECTION ( 'NONE',  ( 0.000000000000000000, 0.000000000000000000, 1.000000000000000000 ) ) ;
#19060=CARTESIAN_POINT ( 'NONE',  ( -2.066987300000001415, 63.14382582708705627, 45.00000000109246656 ) ) ;
#19081=CARTESIAN_POINT ( 'NONE',  ( 2.066987300000001415, 64.00000000000000000, 47.75000000109246656 ) ) ;
#19087=EDGE_LOOP ( 'NONE', ( #12340, #17951, #8116, #3046 ) ) ;
#19090=SURFACE_STYLE_USAGE ( .BOTH. , #12017 ) ;
#19098=CARTESIAN_POINT ( 'NONE',  ( -1.530808498934192803E-16, 66.50000000000000000, 44.30000000218494449 ) ) ;
#19104=ORIENTED_EDGE ( 'NONE', *, *, #2927, .F. ) ;
#19109=CARTESIAN_POINT ( 'NONE',  ( 0.8561741729129472844, 61.93301270000000613, 45.00000000109246656 ) ) ;
#19112=CARTESIAN_POINT ( 'NONE',  ( -1.767766952966369765, 62.23223304703363112, 49.29999999999999716 ) ) ;
#19115=ORIENTED_EDGE ( 'NONE', *, *, #14948, .T. ) ;
#19137=PRODUCT_CONTEXT ( 'NONE', #15093, 'mechanical' ) ;
#19163=CARTESIAN_POINT ( 'NONE',  ( -1.767766952966370209, 65.76776695296638309, 46.69999999999999574 ) ) ;
#19181=CARTESIAN_POINT ( 'NONE',  ( 2.066987300000001415, 64.85617417291294373, 47.80000000109247082 ) ) ;
#19195=CARTESIAN_POINT ( 'NONE',  ( 0.8561741729129460632, 66.06698729999999387, 48.50000000109246656 ) ) ;
#19205=CARTESIAN_POINT ( 'NONE',  ( -1.461580736456473462, 62.53841926354353120, 47.45000000109246230 ) ) ;
#19209=DIRECTION ( 'NONE',  ( 0.000000000000000000, 1.000000000000000000, 0.000000000000000000 ) ) ;
#19260=CARTESIAN_POINT ( 'NONE',  ( -1.530808498934192803E-16, 66.50000000000000000, 47.39999999999999858 ) ) ;
#19268=CARTESIAN_POINT ( 'NONE',  ( -2.156160770143801475, 64.48039283663632659, 45.00000000000000000 ) ) ;
#19278=CARTESIAN_POINT ( 'NONE',  ( 2.499999999999992895, 65.03553390593273775, 49.64999999999998437 ) ) ;
#19292=CARTESIAN_POINT ( 'NONE',  ( 1.035533905932739751, 61.50000000000000000, 48.75000000218494023 ) ) ;
#19294=( BOUNDED_CURVE ( )  B_SPLINE_CURVE ( 2, ( #8337, #701, #7116, #3827, #14567, #17167, #4185, #14025, #11257, #10243, #14662, #5299, #5126, #9702, #15787, #8250, #1234, #14219, #2802, #10138, #3728, #12559, #17076, #4283, #13081, #17704, #786, #13188, #6773, #16230, #12738, #597, #17260, #8154, #15695, #7216, #9794, #14127, #16137, #19181, #19081, #1139, #18558, #11079, #18734, #9610, #5749, #12648, #2353, #5652, #3639, #15596, #11616, #11711, #2165, #17608, #2705, #6590, #18647, #2264, #5214, #11168, #3094, #14864, #1642, #18007, #9078, #11918, #18104, #8777, #6049, #4787, #3203, #69, #13486, #1731, #10437, #7614, #4483, #5947, #7510, #1437, #10634, #10736, #12007, #13578, #4580, #17807, #2996, #8975, #161, #10538, #6147, #17913, #14770, #16732, #16529 ),
 .UNSPECIFIED., .F., .F. ) 
 B_SPLINE_CURVE_WITH_KNOTS ( ( 3, 2, 2, 2, 2, 2, 2, 2, 2, 2, 2, 2, 2, 2, 2, 2, 2, 2, 2, 2, 2, 2, 2, 2, 2, 2, 2, 2, 2, 2, 2, 2, 2, 2, 2, 2, 2, 2, 2, 2, 2, 2, 2, 2, 2, 2, 2, 2, 3 ),
 ( 0.000000000000000000, 0.01785714285714285615, 0.03571428571428571230, 0.05357142857142856845, 0.07142857142857142461, 0.08928571428571430157, 0.1071428571428571369, 0.1250000000000000000, 0.1428571428571428492, 0.1607142857142857262, 0.1785714285714286031, 0.1964285714285713969, 0.2142857142857142738, 0.2321428571428571508, 0.2500000000000000000, 0.2678571428571428492, 0.2857142857142856984, 0.3035714285714285476, 0.3214285714285714524, 0.3392857142857143016, 0.3571428571428572063, 0.3750000000000000000, 0.3928571428571427937, 0.4107142857142856984, 0.4285714285714285476, 0.4464285714285714524, 0.4642857142857143016, 0.4821428571428572063, 0.5000000000000000000, 0.5178571428571429047, 0.5357142857142856984, 0.5535714285714286031, 0.5714285714285713969, 0.5892857142857143016, 0.6071428571428570953, 0.6250000000000001110, 0.6428571428571429047, 0.6607142857142856984, 0.6785714285714286031, 0.6964285714285713969, 0.7142857142857144126, 0.7321428571428570953, 0.7500000000000000000, 0.7678571428571429047, 0.7857142857142855874, 0.8035714285714286031, 0.8214285714285713969, 0.8392857142857143016, 0.8482142859019456971 ),
 .UNSPECIFIED. ) 
 CURVE ( )  GEOMETRIC_REPRESENTATION_ITEM ( )  RATIONAL_B_SPLINE_CURVE ( ( 1.000000000000000000, 0.9238795325112867385, 1.000000000000000000, 0.9238795325112867385, 1.000000000000000000, 0.9238795325112867385, 1.000000000000000000, 0.9238795325112867385, 1.000000000000000000, 0.9238795325112867385, 1.000000000000000000, 0.9238795325112867385, 1.000000000000000000, 0.9238795325112867385, 1.000000000000000000, 0.9238795325112867385, 1.000000000000000000, 0.9238795325112867385, 1.000000000000000000, 0.9238795325112867385, 1.000000000000000000, 0.9238795325112867385, 1.000000000000000000, 0.9238795325112867385, 1.000000000000000000, 0.9238795325112867385, 1.000000000000000000, 0.9238795325112867385, 1.000000000000000000, 0.9238795325112867385, 1.000000000000000000, 0.9238795325112867385, 1.000000000000000000, 0.9238795325112867385, 1.000000000000000000, 0.9238795325112867385, 1.000000000000000000, 0.9238795325112867385, 1.000000000000000000, 0.9238795325112867385, 1.000000000000000000, 0.9238795325112867385, 1.000000000000000000, 0.9238795325112867385, 1.000000000000000000, 0.9238795325112867385, 1.000000000000000000, 0.9238795325112867385, 1.000000000000000000, 0.9238795325112867385, 1.000000000000000000, 0.9238795325112867385, 1.000000000000000000, 0.9238795325112867385, 1.000000000000000000, 0.9238795325112867385, 1.000000000000000000, 0.9238795325112867385, 1.000000000000000000, 0.9238795325112867385, 1.000000000000000000, 0.9238795325112867385, 1.000000000000000000, 0.9238795325112867385, 1.000000000000000000, 0.9238795325112867385, 1.000000000000000000, 0.9238795325112867385, 1.000000000000000000, 0.9238795325112867385, 1.000000000000000000, 0.9238795325112867385, 1.000000000000000000, 0.9238795325112867385, 1.000000000000000000, 0.9238795325112867385, 1.000000000000000000, 0.9238795325112867385, 1.000000000000000000, 0.9238795325112867385, 1.000000000000000000, 0.9238795325112867385, 1.000000000000000000, 0.9238795325112867385, 1.000000000000000000, 0.9238795325112867385, 1.000000000000000000, 0.9238795325112867385, 1.000000000000000000, 0.9238795325112867385, 1.000000000000000000, 0.9238795325112867385, 1.000000000000000000, 0.9238795325112867385, 1.000000000000000000, 0.9619397654556964827, 0.9619397662556434803 ) ) 
 REPRESENTATION_ITEM ( '' )  );
#19296=CARTESIAN_POINT ( 'NONE',  ( -2.066987300000001859, 64.85617417291294373, 49.50000000109246656 ) ) ;
#19305=CARTESIAN_POINT ( 'NONE',  ( -1.461580736456473906, 65.46158073645646880, 48.05000000109247082 ) ) ;
#19318=EDGE_CURVE ( 'NONE', #5104, #17515, #17290, .T. ) ;
#19357=CARTESIAN_POINT ( 'NONE',  ( -2.500000000000001776, 64.00000000000000000, 46.79999999999999716 ) ) ;
#19359=ORIENTED_EDGE ( 'NONE', *, *, #4892, .T. ) ;
#19363=CARTESIAN_POINT ( 'NONE',  ( -2.125375761220501758, 64.66924286904182395, 45.00000000000002842 ) ) ;
#19380=ORIENTED_EDGE ( 'NONE', *, *, #4509, .T. ) ;
#19390=CARTESIAN_POINT ( 'NONE',  ( -2.500000000000000888, 62.96446609406726935, 44.55000000218495870 ) ) ;
ENDSEC;
END-ISO-10303-21;
